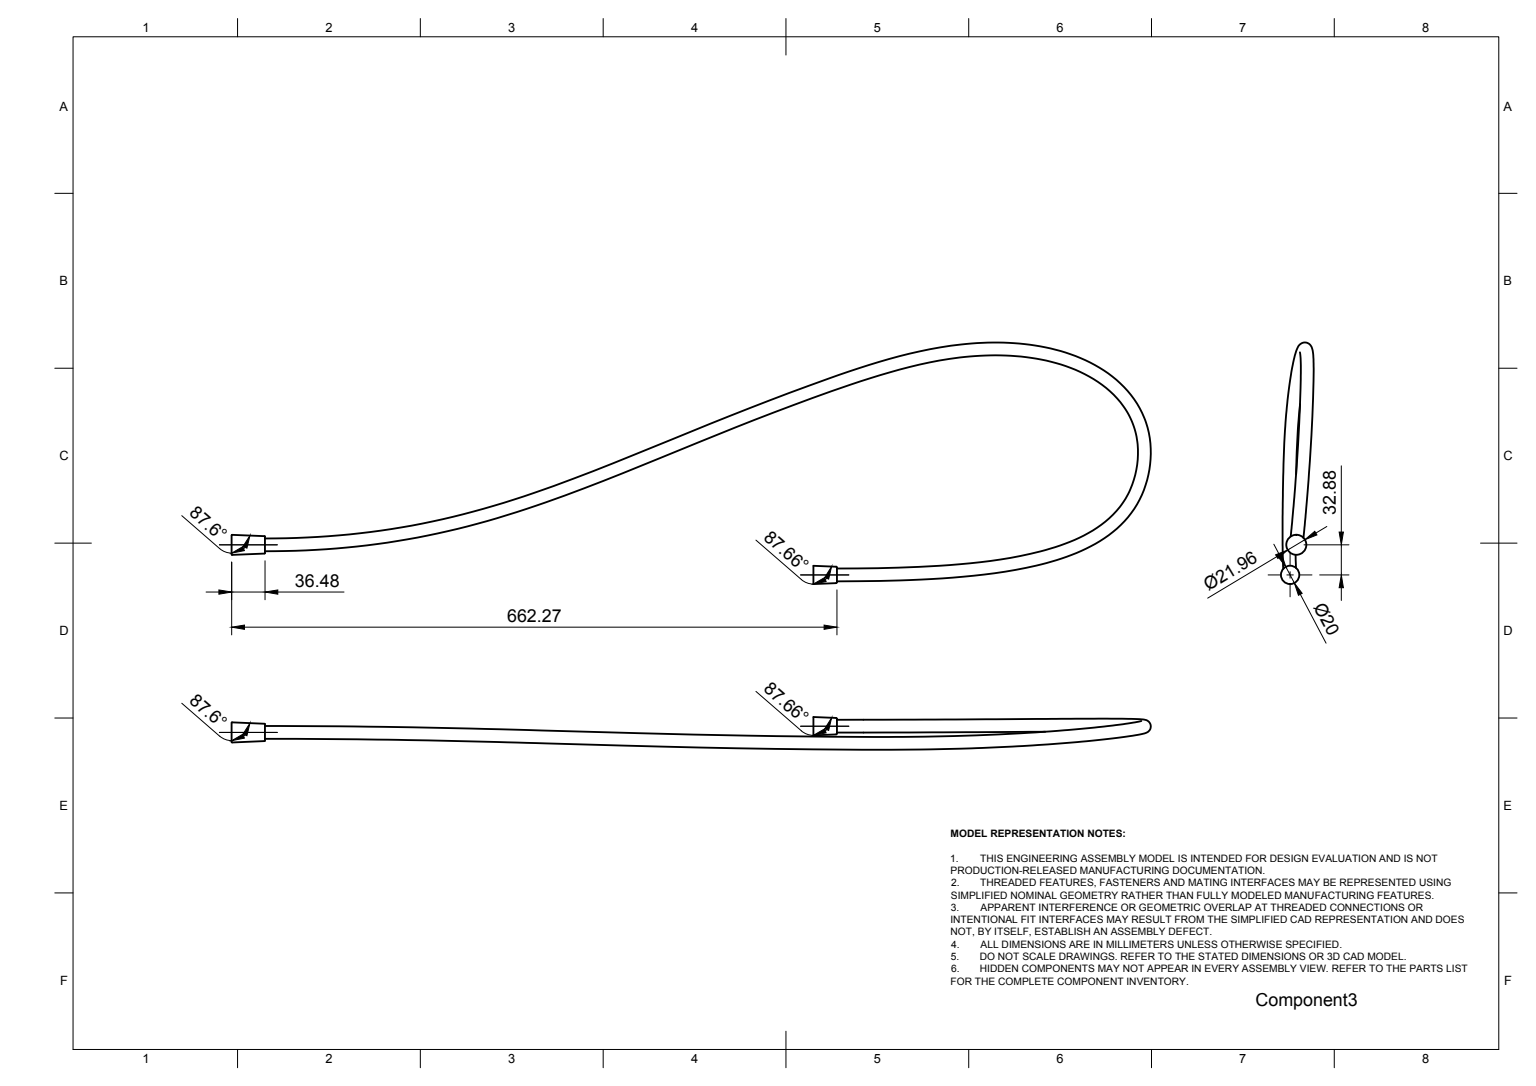
ISO-10303-21;
HEADER;
/* Generated by software containing ST-Developer
 * from STEP Tools, Inc. (www.steptools.com) 
 */

FILE_DESCRIPTION(
/* description */ ('STEP AP214'),
/* implementation_level */ '2;1');

FILE_NAME(
/* name */ 'Component3.step',
/* time_stamp */ '2026-10-06T11:02:40-07:00',
/* author */ (''),
/* organization */ (''),
/* preprocessor_version */ 'ST-DEVELOPER v20.2',
/* originating_system */ 'Autodesk Translation Framework v15.15.0.0',
/* authorisation */ '');

FILE_SCHEMA (('AUTOMOTIVE_DESIGN { 1 0 10303 214 3 1 1 }'));
ENDSEC;

DATA;
#10=MECHANICAL_DESIGN_GEOMETRIC_PRESENTATION_REPRESENTATION('',(#2938),#130910);
#76=CONICAL_SURFACE('',#48147,9.47320447306899,0.0418325464020223);
#77=CONICAL_SURFACE('',#48154,8.94802844775792,0.0407936828678657);
#715=FACE_BOUND('',#14926,.T.);
#716=FACE_BOUND('',#14930,.T.);
#1605=(
BOUNDED_SURFACE()
B_SPLINE_SURFACE(3,3,((#85020,#85021,#85022,#85023,#85024,#85025,#85026,
#85027,#85028,#85029,#85030,#85031,#85032,#85033,#85034,#85035,#85036,#85037,
#85038,#85039,#85040,#85041,#85042,#85043,#85044,#85045,#85046,#85047,#85048,
#85049,#85050,#85051,#85052,#85053,#85054,#85055,#85056,#85057,#85058,#85059,
#85060,#85061,#85062,#85063,#85064,#85065,#85066,#85067,#85068,#85069,#85070,
#85071,#85072,#85073),(#85074,#85075,#85076,#85077,#85078,#85079,#85080,
#85081,#85082,#85083,#85084,#85085,#85086,#85087,#85088,#85089,#85090,#85091,
#85092,#85093,#85094,#85095,#85096,#85097,#85098,#85099,#85100,#85101,#85102,
#85103,#85104,#85105,#85106,#85107,#85108,#85109,#85110,#85111,#85112,#85113,
#85114,#85115,#85116,#85117,#85118,#85119,#85120,#85121,#85122,#85123,#85124,
#85125,#85126,#85127),(#85128,#85129,#85130,#85131,#85132,#85133,#85134,
#85135,#85136,#85137,#85138,#85139,#85140,#85141,#85142,#85143,#85144,#85145,
#85146,#85147,#85148,#85149,#85150,#85151,#85152,#85153,#85154,#85155,#85156,
#85157,#85158,#85159,#85160,#85161,#85162,#85163,#85164,#85165,#85166,#85167,
#85168,#85169,#85170,#85171,#85172,#85173,#85174,#85175,#85176,#85177,#85178,
#85179,#85180,#85181),(#85182,#85183,#85184,#85185,#85186,#85187,#85188,
#85189,#85190,#85191,#85192,#85193,#85194,#85195,#85196,#85197,#85198,#85199,
#85200,#85201,#85202,#85203,#85204,#85205,#85206,#85207,#85208,#85209,#85210,
#85211,#85212,#85213,#85214,#85215,#85216,#85217,#85218,#85219,#85220,#85221,
#85222,#85223,#85224,#85225,#85226,#85227,#85228,#85229,#85230,#85231,#85232,
#85233,#85234,#85235),(#85236,#85237,#85238,#85239,#85240,#85241,#85242,
#85243,#85244,#85245,#85246,#85247,#85248,#85249,#85250,#85251,#85252,#85253,
#85254,#85255,#85256,#85257,#85258,#85259,#85260,#85261,#85262,#85263,#85264,
#85265,#85266,#85267,#85268,#85269,#85270,#85271,#85272,#85273,#85274,#85275,
#85276,#85277,#85278,#85279,#85280,#85281,#85282,#85283,#85284,#85285,#85286,
#85287,#85288,#85289),(#85290,#85291,#85292,#85293,#85294,#85295,#85296,
#85297,#85298,#85299,#85300,#85301,#85302,#85303,#85304,#85305,#85306,#85307,
#85308,#85309,#85310,#85311,#85312,#85313,#85314,#85315,#85316,#85317,#85318,
#85319,#85320,#85321,#85322,#85323,#85324,#85325,#85326,#85327,#85328,#85329,
#85330,#85331,#85332,#85333,#85334,#85335,#85336,#85337,#85338,#85339,#85340,
#85341,#85342,#85343),(#85344,#85345,#85346,#85347,#85348,#85349,#85350,
#85351,#85352,#85353,#85354,#85355,#85356,#85357,#85358,#85359,#85360,#85361,
#85362,#85363,#85364,#85365,#85366,#85367,#85368,#85369,#85370,#85371,#85372,
#85373,#85374,#85375,#85376,#85377,#85378,#85379,#85380,#85381,#85382,#85383,
#85384,#85385,#85386,#85387,#85388,#85389,#85390,#85391,#85392,#85393,#85394,
#85395,#85396,#85397)),.UNSPECIFIED.,.T.,.F.,.F.)
B_SPLINE_SURFACE_WITH_KNOTS((4,3,4),(4,2,2,2,2,2,2,2,2,2,2,2,2,2,2,2,2,
2,2,2,2,2,2,2,2,2,4),(0.,0.5,1.),(0.,0.00855967103632646,0.0171193420726529,
0.0342386841453058,0.0684773682906117,0.136954736581223,0.171193420726529,
0.205432104871835,0.239670789017141,0.273909473162447,0.302569805907928,
0.316899972280669,0.324065055467039,0.33123013865341,0.358116418237434,
0.385002697821458,0.438775256989507,0.492547816157555,0.546320375325604,
0.555016077087237,0.563711778848869,0.581103182372135,0.615885989418665,
0.711914492063999,0.807942994709333,0.903971497354666,1.),.UNSPECIFIED.)
GEOMETRIC_REPRESENTATION_ITEM()
RATIONAL_B_SPLINE_SURFACE(((1.,1.,1.,1.,1.,1.,1.,1.,1.,1.,1.,1.,1.,1.,1.,
1.,1.,1.,1.,1.,1.,1.,1.,1.,1.,1.,1.,1.,1.,1.,1.,1.,1.,1.,1.,1.,1.,1.,1.,
1.,1.,1.,1.,1.,1.,1.,1.,1.,1.,1.,1.,1.,1.,1.),(0.333333333333333,0.333333333333333,
0.333333333333333,0.333333333333333,0.333333333333333,0.333333333333333,
0.333333333333333,0.333333333333333,0.333333333333333,0.333333333333333,
0.333333333333333,0.333333333333333,0.333333333333333,0.333333333333333,
0.333333333333333,0.333333333333333,0.333333333333333,0.333333333333333,
0.333333333333333,0.333333333333333,0.333333333333333,0.333333333333333,
0.333333333333333,0.333333333333333,0.333333333333333,0.333333333333333,
0.333333333333333,0.333333333333333,0.333333333333333,0.333333333333333,
0.333333333333333,0.333333333333333,0.333333333333333,0.333333333333333,
0.333333333333333,0.333333333333333,0.333333333333333,0.333333333333333,
0.333333333333333,0.333333333333333,0.333333333333333,0.333333333333333,
0.333333333333333,0.333333333333333,0.333333333333333,0.333333333333333,
0.333333333333333,0.333333333333333,0.333333333333333,0.333333333333333,
0.333333333333333,0.333333333333333,0.333333333333333,0.333333333333333),
(0.333333333333333,0.333333333333333,0.333333333333333,0.333333333333333,
0.333333333333333,0.333333333333333,0.333333333333333,0.333333333333333,
0.333333333333333,0.333333333333333,0.333333333333333,0.333333333333333,
0.333333333333333,0.333333333333333,0.333333333333333,0.333333333333333,
0.333333333333333,0.333333333333333,0.333333333333333,0.333333333333333,
0.333333333333333,0.333333333333333,0.333333333333333,0.333333333333333,
0.333333333333333,0.333333333333333,0.333333333333333,0.333333333333333,
0.333333333333333,0.333333333333333,0.333333333333333,0.333333333333333,
0.333333333333333,0.333333333333333,0.333333333333333,0.333333333333333,
0.333333333333333,0.333333333333333,0.333333333333333,0.333333333333333,
0.333333333333333,0.333333333333333,0.333333333333333,0.333333333333333,
0.333333333333333,0.333333333333333,0.333333333333333,0.333333333333333,
0.333333333333333,0.333333333333333,0.333333333333333,0.333333333333333,
0.333333333333333,0.333333333333333),(1.,1.,1.,1.,1.,1.,1.,1.,1.,1.,1.,
1.,1.,1.,1.,1.,1.,1.,1.,1.,1.,1.,1.,1.,1.,1.,1.,1.,1.,1.,1.,1.,1.,1.,1.,
1.,1.,1.,1.,1.,1.,1.,1.,1.,1.,1.,1.,1.,1.,1.,1.,1.,1.,1.),(0.333333333333333,
0.333333333333333,0.333333333333333,0.333333333333333,0.333333333333333,
0.333333333333333,0.333333333333333,0.333333333333333,0.333333333333333,
0.333333333333333,0.333333333333333,0.333333333333333,0.333333333333333,
0.333333333333333,0.333333333333333,0.333333333333333,0.333333333333333,
0.333333333333333,0.333333333333333,0.333333333333333,0.333333333333333,
0.333333333333333,0.333333333333333,0.333333333333333,0.333333333333333,
0.333333333333333,0.333333333333333,0.333333333333333,0.333333333333333,
0.333333333333333,0.333333333333333,0.333333333333333,0.333333333333333,
0.333333333333333,0.333333333333333,0.333333333333333,0.333333333333333,
0.333333333333333,0.333333333333333,0.333333333333333,0.333333333333333,
0.333333333333333,0.333333333333333,0.333333333333333,0.333333333333333,
0.333333333333333,0.333333333333333,0.333333333333333,0.333333333333333,
0.333333333333333,0.333333333333333,0.333333333333333,0.333333333333333,
0.333333333333333),(0.333333333333333,0.333333333333333,0.333333333333333,
0.333333333333333,0.333333333333333,0.333333333333333,0.333333333333333,
0.333333333333333,0.333333333333333,0.333333333333333,0.333333333333333,
0.333333333333333,0.333333333333333,0.333333333333333,0.333333333333333,
0.333333333333333,0.333333333333333,0.333333333333333,0.333333333333333,
0.333333333333333,0.333333333333333,0.333333333333333,0.333333333333333,
0.333333333333333,0.333333333333333,0.333333333333333,0.333333333333333,
0.333333333333333,0.333333333333333,0.333333333333333,0.333333333333333,
0.333333333333333,0.333333333333333,0.333333333333333,0.333333333333333,
0.333333333333333,0.333333333333333,0.333333333333333,0.333333333333333,
0.333333333333333,0.333333333333333,0.333333333333333,0.333333333333333,
0.333333333333333,0.333333333333333,0.333333333333333,0.333333333333333,
0.333333333333333,0.333333333333333,0.333333333333333,0.333333333333333,
0.333333333333333,0.333333333333333,0.333333333333333),(1.,1.,1.,1.,1.,
1.,1.,1.,1.,1.,1.,1.,1.,1.,1.,1.,1.,1.,1.,1.,1.,1.,1.,1.,1.,1.,1.,1.,1.,
1.,1.,1.,1.,1.,1.,1.,1.,1.,1.,1.,1.,1.,1.,1.,1.,1.,1.,1.,1.,1.,1.,1.,1.,
1.)))
REPRESENTATION_ITEM('')
SURFACE()
);
#1606=(
BOUNDED_SURFACE()
B_SPLINE_SURFACE(3,3,((#85525,#85526,#85527,#85528,#85529,#85530,#85531,
#85532,#85533,#85534,#85535,#85536,#85537,#85538,#85539,#85540,#85541,#85542,
#85543,#85544,#85545,#85546,#85547,#85548,#85549,#85550,#85551,#85552,#85553,
#85554,#85555,#85556,#85557,#85558,#85559,#85560,#85561,#85562,#85563,#85564,
#85565,#85566,#85567,#85568,#85569,#85570,#85571,#85572,#85573,#85574,#85575,
#85576,#85577,#85578),(#85579,#85580,#85581,#85582,#85583,#85584,#85585,
#85586,#85587,#85588,#85589,#85590,#85591,#85592,#85593,#85594,#85595,#85596,
#85597,#85598,#85599,#85600,#85601,#85602,#85603,#85604,#85605,#85606,#85607,
#85608,#85609,#85610,#85611,#85612,#85613,#85614,#85615,#85616,#85617,#85618,
#85619,#85620,#85621,#85622,#85623,#85624,#85625,#85626,#85627,#85628,#85629,
#85630,#85631,#85632),(#85633,#85634,#85635,#85636,#85637,#85638,#85639,
#85640,#85641,#85642,#85643,#85644,#85645,#85646,#85647,#85648,#85649,#85650,
#85651,#85652,#85653,#85654,#85655,#85656,#85657,#85658,#85659,#85660,#85661,
#85662,#85663,#85664,#85665,#85666,#85667,#85668,#85669,#85670,#85671,#85672,
#85673,#85674,#85675,#85676,#85677,#85678,#85679,#85680,#85681,#85682,#85683,
#85684,#85685,#85686),(#85687,#85688,#85689,#85690,#85691,#85692,#85693,
#85694,#85695,#85696,#85697,#85698,#85699,#85700,#85701,#85702,#85703,#85704,
#85705,#85706,#85707,#85708,#85709,#85710,#85711,#85712,#85713,#85714,#85715,
#85716,#85717,#85718,#85719,#85720,#85721,#85722,#85723,#85724,#85725,#85726,
#85727,#85728,#85729,#85730,#85731,#85732,#85733,#85734,#85735,#85736,#85737,
#85738,#85739,#85740),(#85741,#85742,#85743,#85744,#85745,#85746,#85747,
#85748,#85749,#85750,#85751,#85752,#85753,#85754,#85755,#85756,#85757,#85758,
#85759,#85760,#85761,#85762,#85763,#85764,#85765,#85766,#85767,#85768,#85769,
#85770,#85771,#85772,#85773,#85774,#85775,#85776,#85777,#85778,#85779,#85780,
#85781,#85782,#85783,#85784,#85785,#85786,#85787,#85788,#85789,#85790,#85791,
#85792,#85793,#85794),(#85795,#85796,#85797,#85798,#85799,#85800,#85801,
#85802,#85803,#85804,#85805,#85806,#85807,#85808,#85809,#85810,#85811,#85812,
#85813,#85814,#85815,#85816,#85817,#85818,#85819,#85820,#85821,#85822,#85823,
#85824,#85825,#85826,#85827,#85828,#85829,#85830,#85831,#85832,#85833,#85834,
#85835,#85836,#85837,#85838,#85839,#85840,#85841,#85842,#85843,#85844,#85845,
#85846,#85847,#85848),(#85849,#85850,#85851,#85852,#85853,#85854,#85855,
#85856,#85857,#85858,#85859,#85860,#85861,#85862,#85863,#85864,#85865,#85866,
#85867,#85868,#85869,#85870,#85871,#85872,#85873,#85874,#85875,#85876,#85877,
#85878,#85879,#85880,#85881,#85882,#85883,#85884,#85885,#85886,#85887,#85888,
#85889,#85890,#85891,#85892,#85893,#85894,#85895,#85896,#85897,#85898,#85899,
#85900,#85901,#85902)),.UNSPECIFIED.,.T.,.F.,.F.)
B_SPLINE_SURFACE_WITH_KNOTS((4,3,4),(4,2,2,2,2,2,2,2,2,2,2,2,2,2,2,2,2,
2,2,2,2,2,2,2,2,2,4),(0.,0.5,1.),(0.,0.00855967103632646,0.0171193420726529,
0.0342386841453058,0.0684773682906117,0.136954736581223,0.171193420726529,
0.205432104871835,0.239670789017141,0.273909473162447,0.302569805907928,
0.316899972280669,0.324065055467039,0.33123013865341,0.358116418237434,
0.385002697821458,0.438775256989507,0.492547816157555,0.546320375325604,
0.555016077087237,0.563711778848869,0.581103182372135,0.615885989418665,
0.711914492063999,0.807942994709333,0.903971497354666,1.),.UNSPECIFIED.)
GEOMETRIC_REPRESENTATION_ITEM()
RATIONAL_B_SPLINE_SURFACE(((1.,1.,1.,1.,1.,1.,1.,1.,1.,1.,1.,1.,1.,1.,1.,
1.,1.,1.,1.,1.,1.,1.,1.,1.,1.,1.,1.,1.,1.,1.,1.,1.,1.,1.,1.,1.,1.,1.,1.,
1.,1.,1.,1.,1.,1.,1.,1.,1.,1.,1.,1.,1.,1.,1.),(0.333333333333333,0.333333333333333,
0.333333333333333,0.333333333333333,0.333333333333333,0.333333333333333,
0.333333333333333,0.333333333333333,0.333333333333333,0.333333333333333,
0.333333333333333,0.333333333333333,0.333333333333333,0.333333333333333,
0.333333333333333,0.333333333333333,0.333333333333333,0.333333333333333,
0.333333333333333,0.333333333333333,0.333333333333333,0.333333333333333,
0.333333333333333,0.333333333333333,0.333333333333333,0.333333333333333,
0.333333333333333,0.333333333333333,0.333333333333333,0.333333333333333,
0.333333333333333,0.333333333333333,0.333333333333333,0.333333333333333,
0.333333333333333,0.333333333333333,0.333333333333333,0.333333333333333,
0.333333333333333,0.333333333333333,0.333333333333333,0.333333333333333,
0.333333333333333,0.333333333333333,0.333333333333333,0.333333333333333,
0.333333333333333,0.333333333333333,0.333333333333333,0.333333333333333,
0.333333333333333,0.333333333333333,0.333333333333333,0.333333333333333),
(0.333333333333333,0.333333333333333,0.333333333333333,0.333333333333333,
0.333333333333333,0.333333333333333,0.333333333333333,0.333333333333333,
0.333333333333333,0.333333333333333,0.333333333333333,0.333333333333333,
0.333333333333333,0.333333333333333,0.333333333333333,0.333333333333333,
0.333333333333333,0.333333333333333,0.333333333333333,0.333333333333333,
0.333333333333333,0.333333333333333,0.333333333333333,0.333333333333333,
0.333333333333333,0.333333333333333,0.333333333333333,0.333333333333333,
0.333333333333333,0.333333333333333,0.333333333333333,0.333333333333333,
0.333333333333333,0.333333333333333,0.333333333333333,0.333333333333333,
0.333333333333333,0.333333333333333,0.333333333333333,0.333333333333333,
0.333333333333333,0.333333333333333,0.333333333333333,0.333333333333333,
0.333333333333333,0.333333333333333,0.333333333333333,0.333333333333333,
0.333333333333333,0.333333333333333,0.333333333333333,0.333333333333333,
0.333333333333333,0.333333333333333),(1.,1.,1.,1.,1.,1.,1.,1.,1.,1.,1.,
1.,1.,1.,1.,1.,1.,1.,1.,1.,1.,1.,1.,1.,1.,1.,1.,1.,1.,1.,1.,1.,1.,1.,1.,
1.,1.,1.,1.,1.,1.,1.,1.,1.,1.,1.,1.,1.,1.,1.,1.,1.,1.,1.),(0.333333333333333,
0.333333333333333,0.333333333333333,0.333333333333333,0.333333333333333,
0.333333333333333,0.333333333333333,0.333333333333333,0.333333333333333,
0.333333333333333,0.333333333333333,0.333333333333333,0.333333333333333,
0.333333333333333,0.333333333333333,0.333333333333333,0.333333333333333,
0.333333333333333,0.333333333333333,0.333333333333333,0.333333333333333,
0.333333333333333,0.333333333333333,0.333333333333333,0.333333333333333,
0.333333333333333,0.333333333333333,0.333333333333333,0.333333333333333,
0.333333333333333,0.333333333333333,0.333333333333333,0.333333333333333,
0.333333333333333,0.333333333333333,0.333333333333333,0.333333333333333,
0.333333333333333,0.333333333333333,0.333333333333333,0.333333333333333,
0.333333333333333,0.333333333333333,0.333333333333333,0.333333333333333,
0.333333333333333,0.333333333333333,0.333333333333333,0.333333333333333,
0.333333333333333,0.333333333333333,0.333333333333333,0.333333333333333,
0.333333333333333),(0.333333333333333,0.333333333333333,0.333333333333333,
0.333333333333333,0.333333333333333,0.333333333333333,0.333333333333333,
0.333333333333333,0.333333333333333,0.333333333333333,0.333333333333333,
0.333333333333333,0.333333333333333,0.333333333333333,0.333333333333333,
0.333333333333333,0.333333333333333,0.333333333333333,0.333333333333333,
0.333333333333333,0.333333333333333,0.333333333333333,0.333333333333333,
0.333333333333333,0.333333333333333,0.333333333333333,0.333333333333333,
0.333333333333333,0.333333333333333,0.333333333333333,0.333333333333333,
0.333333333333333,0.333333333333333,0.333333333333333,0.333333333333333,
0.333333333333333,0.333333333333333,0.333333333333333,0.333333333333333,
0.333333333333333,0.333333333333333,0.333333333333333,0.333333333333333,
0.333333333333333,0.333333333333333,0.333333333333333,0.333333333333333,
0.333333333333333,0.333333333333333,0.333333333333333,0.333333333333333,
0.333333333333333,0.333333333333333,0.333333333333333),(1.,1.,1.,1.,1.,
1.,1.,1.,1.,1.,1.,1.,1.,1.,1.,1.,1.,1.,1.,1.,1.,1.,1.,1.,1.,1.,1.,1.,1.,
1.,1.,1.,1.,1.,1.,1.,1.,1.,1.,1.,1.,1.,1.,1.,1.,1.,1.,1.,1.,1.,1.,1.,1.,
1.)))
REPRESENTATION_ITEM('')
SURFACE()
);
#2186=B_SPLINE_CURVE_WITH_KNOTS('',3,(#85402,#85403,#85404,#85405,#85406,
#85407,#85408,#85409,#85410,#85411,#85412,#85413,#85414,#85415,#85416,#85417,
#85418,#85419,#85420,#85421,#85422,#85423,#85424,#85425,#85426,#85427,#85428,
#85429,#85430,#85431,#85432,#85433,#85434,#85435,#85436,#85437,#85438,#85439,
#85440,#85441,#85442,#85443,#85444,#85445,#85446,#85447,#85448,#85449,#85450,
#85451,#85452,#85453,#85454,#85455),.UNSPECIFIED.,.F.,.F.,(4,2,2,2,2,2,
2,2,2,2,2,2,2,2,2,2,2,2,2,2,2,2,2,2,2,2,4),(0.,0.00855967103632646,0.0171193420726529,
0.0342386841453058,0.0684773682906117,0.136954736581223,0.171193420726529,
0.205432104871835,0.239670789017141,0.273909473162447,0.302569805907928,
0.316899972280669,0.324065055467039,0.33123013865341,0.358116418237434,
0.385002697821458,0.438775256989507,0.492547816157555,0.546320375325604,
0.555016077087237,0.563711778848869,0.581103182372135,0.615885989418665,
0.711914492063999,0.807942994709333,0.903971497354666,1.),.UNSPECIFIED.);
#2187=B_SPLINE_CURVE_WITH_KNOTS('',3,(#85458,#85459,#85460,#85461,#85462,
#85463,#85464,#85465,#85466,#85467,#85468,#85469,#85470,#85471,#85472,#85473,
#85474,#85475,#85476,#85477,#85478,#85479,#85480,#85481,#85482,#85483,#85484,
#85485,#85486,#85487,#85488,#85489,#85490,#85491,#85492,#85493,#85494,#85495,
#85496,#85497,#85498,#85499,#85500,#85501,#85502,#85503,#85504,#85505,#85506,
#85507,#85508,#85509,#85510,#85511),.UNSPECIFIED.,.F.,.F.,(4,2,2,2,2,2,
2,2,2,2,2,2,2,2,2,2,2,2,2,2,2,2,2,2,2,2,4),(0.,0.00855967103632646,0.0171193420726529,
0.0342386841453058,0.0684773682906117,0.136954736581223,0.171193420726529,
0.205432104871835,0.239670789017141,0.273909473162447,0.302569805907928,
0.316899972280669,0.324065055467039,0.33123013865341,0.358116418237434,
0.385002697821458,0.438775256989507,0.492547816157555,0.546320375325604,
0.555016077087237,0.563711778848869,0.581103182372135,0.615885989418665,
0.711914492063999,0.807942994709333,0.903971497354666,1.),.UNSPECIFIED.);
#2922=SHAPE_REPRESENTATION_RELATIONSHIP('SRR','None',#130944,#2930);
#2930=ADVANCED_BREP_SHAPE_REPRESENTATION('',(#2945),#130904);
#2938=STYLED_ITEM('',(#130991),#2945);
#2945=MANIFOLD_SOLID_BREP('Body1',#45452);
#3571=PLANE('',#48156);
#3572=PLANE('',#48157);
#3573=PLANE('',#48160);
#3574=PLANE('',#48161);
#5020=LINE('',#85019,#6794);
#5021=LINE('',#85521,#6795);
#6794=VECTOR('',#57507,9.47320447306899);
#6795=VECTOR('',#57524,8.94802844775792);
#10885=FACE_OUTER_BOUND('',#14918,.T.);
#10886=FACE_OUTER_BOUND('',#14919,.T.);
#10887=FACE_OUTER_BOUND('',#14920,.T.);
#10888=FACE_OUTER_BOUND('',#14921,.T.);
#10889=FACE_OUTER_BOUND('',#14922,.T.);
#10890=FACE_OUTER_BOUND('',#14923,.T.);
#10891=FACE_OUTER_BOUND('',#14924,.T.);
#10892=FACE_OUTER_BOUND('',#14925,.T.);
#10893=FACE_OUTER_BOUND('',#14927,.T.);
#10894=FACE_OUTER_BOUND('',#14928,.T.);
#10895=FACE_OUTER_BOUND('',#14929,.T.);
#14918=EDGE_LOOP('',(#35008,#35009,#35010,#35011,#35012));
#14919=EDGE_LOOP('',(#35013,#35014,#35015,#35016));
#14920=EDGE_LOOP('',(#35017,#35018,#35019,#35020,#35021));
#14921=EDGE_LOOP('',(#35022,#35023,#35024,#35025));
#14922=EDGE_LOOP('',(#35026,#35027,#35028,#35029));
#14923=EDGE_LOOP('',(#35030,#35031,#35032,#35033));
#14924=EDGE_LOOP('',(#35034));
#14925=EDGE_LOOP('',(#35035));
#14926=EDGE_LOOP('',(#35036,#35037));
#14927=EDGE_LOOP('',(#35038,#35039,#35040,#35041));
#14928=EDGE_LOOP('',(#35042));
#14929=EDGE_LOOP('',(#35043));
#14930=EDGE_LOOP('',(#35044,#35045));
#18957=CIRCLE('',#48139,10.9781962809611);
#18958=CIRCLE('',#48140,10.9781962809611);
#18959=CIRCLE('',#48141,0.5);
#18960=CIRCLE('',#48142,10.4786337076502);
#18961=CIRCLE('',#48144,9.49325771931311);
#18962=CIRCLE('',#48145,0.5);
#18963=CIRCLE('',#48146,8.99369514600215);
#18964=CIRCLE('',#48148,6.99999999999999);
#18965=CIRCLE('',#48149,6.99999999999999);
#18966=CIRCLE('',#48151,8.98718018777775);
#18967=CIRCLE('',#48152,1.);
#18968=CIRCLE('',#48153,7.98801213467717);
#18969=CIRCLE('',#48155,10.);
#18970=CIRCLE('',#48158,6.99999999999999);
#18971=CIRCLE('',#48159,6.99999999999999);
#22203=VERTEX_POINT('',#85005);
#22204=VERTEX_POINT('',#85006);
#22205=VERTEX_POINT('',#85009);
#22206=VERTEX_POINT('',#85013);
#22207=VERTEX_POINT('',#85015);
#22208=VERTEX_POINT('',#85398);
#22209=VERTEX_POINT('',#85399);
#22210=VERTEX_POINT('',#85401);
#22211=VERTEX_POINT('',#85456);
#22212=VERTEX_POINT('',#85513);
#22213=VERTEX_POINT('',#85515);
#22214=VERTEX_POINT('',#85519);
#26848=EDGE_CURVE('',#22203,#22204,#18957,.T.);
#26849=EDGE_CURVE('',#22204,#22203,#18958,.T.);
#26850=EDGE_CURVE('',#22204,#22205,#18959,.T.);
#26851=EDGE_CURVE('',#22205,#22205,#18960,.T.);
#26852=EDGE_CURVE('',#22206,#22206,#18961,.T.);
#26853=EDGE_CURVE('',#22206,#22207,#18962,.T.);
#26854=EDGE_CURVE('',#22207,#22207,#18963,.T.);
#26855=EDGE_CURVE('',#22203,#22206,#5020,.T.);
#26856=EDGE_CURVE('',#22208,#22209,#18964,.T.);
#26857=EDGE_CURVE('',#22209,#22210,#2186,.T.);
#26858=EDGE_CURVE('',#22211,#22210,#18965,.T.);
#26859=EDGE_CURVE('',#22208,#22211,#2187,.T.);
#26860=EDGE_CURVE('',#22212,#22212,#18966,.T.);
#26861=EDGE_CURVE('',#22212,#22213,#18967,.T.);
#26862=EDGE_CURVE('',#22213,#22213,#18968,.T.);
#26863=EDGE_CURVE('',#22214,#22214,#18969,.T.);
#26864=EDGE_CURVE('',#22214,#22212,#5021,.T.);
#26865=EDGE_CURVE('',#22209,#22208,#18970,.T.);
#26866=EDGE_CURVE('',#22210,#22211,#18971,.T.);
#35008=ORIENTED_EDGE('',*,*,#26848,.F.);
#35009=ORIENTED_EDGE('',*,*,#26849,.F.);
#35010=ORIENTED_EDGE('',*,*,#26850,.T.);
#35011=ORIENTED_EDGE('',*,*,#26851,.F.);
#35012=ORIENTED_EDGE('',*,*,#26850,.F.);
#35013=ORIENTED_EDGE('',*,*,#26852,.F.);
#35014=ORIENTED_EDGE('',*,*,#26853,.T.);
#35015=ORIENTED_EDGE('',*,*,#26854,.F.);
#35016=ORIENTED_EDGE('',*,*,#26853,.F.);
#35017=ORIENTED_EDGE('',*,*,#26848,.T.);
#35018=ORIENTED_EDGE('',*,*,#26849,.T.);
#35019=ORIENTED_EDGE('',*,*,#26855,.T.);
#35020=ORIENTED_EDGE('',*,*,#26852,.T.);
#35021=ORIENTED_EDGE('',*,*,#26855,.F.);
#35022=ORIENTED_EDGE('',*,*,#26856,.T.);
#35023=ORIENTED_EDGE('',*,*,#26857,.T.);
#35024=ORIENTED_EDGE('',*,*,#26858,.F.);
#35025=ORIENTED_EDGE('',*,*,#26859,.F.);
#35026=ORIENTED_EDGE('',*,*,#26860,.F.);
#35027=ORIENTED_EDGE('',*,*,#26861,.T.);
#35028=ORIENTED_EDGE('',*,*,#26862,.F.);
#35029=ORIENTED_EDGE('',*,*,#26861,.F.);
#35030=ORIENTED_EDGE('',*,*,#26863,.F.);
#35031=ORIENTED_EDGE('',*,*,#26864,.T.);
#35032=ORIENTED_EDGE('',*,*,#26860,.T.);
#35033=ORIENTED_EDGE('',*,*,#26864,.F.);
#35034=ORIENTED_EDGE('',*,*,#26863,.T.);
#35035=ORIENTED_EDGE('',*,*,#26862,.T.);
#35036=ORIENTED_EDGE('',*,*,#26856,.F.);
#35037=ORIENTED_EDGE('',*,*,#26865,.F.);
#35038=ORIENTED_EDGE('',*,*,#26857,.F.);
#35039=ORIENTED_EDGE('',*,*,#26865,.T.);
#35040=ORIENTED_EDGE('',*,*,#26859,.T.);
#35041=ORIENTED_EDGE('',*,*,#26866,.F.);
#35042=ORIENTED_EDGE('',*,*,#26851,.T.);
#35043=ORIENTED_EDGE('',*,*,#26854,.T.);
#35044=ORIENTED_EDGE('',*,*,#26858,.T.);
#35045=ORIENTED_EDGE('',*,*,#26866,.T.);
#41960=TOROIDAL_SURFACE('',#48138,10.4786337076502,0.5);
#41961=TOROIDAL_SURFACE('',#48143,8.99369514600215,0.5);
#41962=TOROIDAL_SURFACE('',#48150,7.98801213467717,1.);
#43465=ADVANCED_FACE('',(#10885),#41960,.T.);
#43466=ADVANCED_FACE('',(#10886),#41961,.T.);
#43467=ADVANCED_FACE('',(#10887),#76,.T.);
#43468=ADVANCED_FACE('',(#10888),#1605,.T.);
#43469=ADVANCED_FACE('',(#10889),#41962,.T.);
#43470=ADVANCED_FACE('',(#10890),#77,.T.);
#43471=ADVANCED_FACE('',(#10891),#3571,.F.);
#43472=ADVANCED_FACE('',(#10892,#715),#3572,.F.);
#43473=ADVANCED_FACE('',(#10893),#1606,.T.);
#43474=ADVANCED_FACE('',(#10894),#3573,.F.);
#43475=ADVANCED_FACE('',(#10895,#716),#3574,.F.);
#45452=CLOSED_SHELL('',(#43465,#43466,#43467,#43468,#43469,#43470,#43471,
#43472,#43473,#43474,#43475));
#48137=AXIS2_PLACEMENT_3D('',#85003,#57485,#57486);
#48138=AXIS2_PLACEMENT_3D('',#85004,#57487,#57488);
#48139=AXIS2_PLACEMENT_3D('',#85007,#57489,#57490);
#48140=AXIS2_PLACEMENT_3D('',#85008,#57491,#57492);
#48141=AXIS2_PLACEMENT_3D('',#85010,#57493,#57494);
#48142=AXIS2_PLACEMENT_3D('',#85011,#57495,#57496);
#48143=AXIS2_PLACEMENT_3D('',#85012,#57497,#57498);
#48144=AXIS2_PLACEMENT_3D('',#85014,#57499,#57500);
#48145=AXIS2_PLACEMENT_3D('',#85016,#57501,#57502);
#48146=AXIS2_PLACEMENT_3D('',#85017,#57503,#57504);
#48147=AXIS2_PLACEMENT_3D('',#85018,#57505,#57506);
#48148=AXIS2_PLACEMENT_3D('',#85400,#57508,#57509);
#48149=AXIS2_PLACEMENT_3D('',#85457,#57510,#57511);
#48150=AXIS2_PLACEMENT_3D('',#85512,#57512,#57513);
#48151=AXIS2_PLACEMENT_3D('',#85514,#57514,#57515);
#48152=AXIS2_PLACEMENT_3D('',#85516,#57516,#57517);
#48153=AXIS2_PLACEMENT_3D('',#85517,#57518,#57519);
#48154=AXIS2_PLACEMENT_3D('',#85518,#57520,#57521);
#48155=AXIS2_PLACEMENT_3D('',#85520,#57522,#57523);
#48156=AXIS2_PLACEMENT_3D('',#85522,#57525,#57526);
#48157=AXIS2_PLACEMENT_3D('',#85523,#57527,#57528);
#48158=AXIS2_PLACEMENT_3D('',#85524,#57529,#57530);
#48159=AXIS2_PLACEMENT_3D('',#85903,#57531,#57532);
#48160=AXIS2_PLACEMENT_3D('',#85904,#57533,#57534);
#48161=AXIS2_PLACEMENT_3D('',#85905,#57535,#57536);
#57485=DIRECTION('axis',(0.,0.,1.));
#57486=DIRECTION('refdir',(1.,0.,0.));
#57487=DIRECTION('center_axis',(0.,-1.,0.));
#57488=DIRECTION('ref_axis',(0.,0.,-1.));
#57489=DIRECTION('center_axis',(0.,-1.,0.));
#57490=DIRECTION('ref_axis',(0.,0.,-1.));
#57491=DIRECTION('center_axis',(0.,-1.,0.));
#57492=DIRECTION('ref_axis',(0.,0.,-1.));
#57493=DIRECTION('center_axis',(-1.,0.,0.));
#57494=DIRECTION('ref_axis',(0.,0.,1.));
#57495=DIRECTION('center_axis',(0.,1.,0.));
#57496=DIRECTION('ref_axis',(0.,0.,-1.));
#57497=DIRECTION('center_axis',(0.,1.,0.));
#57498=DIRECTION('ref_axis',(0.,0.,1.));
#57499=DIRECTION('center_axis',(0.,1.,0.));
#57500=DIRECTION('ref_axis',(0.,0.,-1.));
#57501=DIRECTION('center_axis',(-1.,0.,0.));
#57502=DIRECTION('ref_axis',(0.,0.,-1.));
#57503=DIRECTION('center_axis',(0.,-1.,0.));
#57504=DIRECTION('ref_axis',(0.,0.,1.));
#57505=DIRECTION('center_axis',(0.,1.,0.));
#57506=DIRECTION('ref_axis',(0.,0.,1.));
#57507=DIRECTION('',(5.12151535729607E-18,-0.999125146621934,0.041820346575534));
#57508=DIRECTION('center_axis',(0.,-1.,0.));
#57509=DIRECTION('ref_axis',(0.,0.,-1.));
#57510=DIRECTION('center_axis',(8.61122783338974E-15,1.,9.154793709916E-16));
#57511=DIRECTION('ref_axis',(0.161066048973386,-4.83449910768251E-16,-0.986943629529115));
#57512=DIRECTION('center_axis',(0.,1.,0.));
#57513=DIRECTION('ref_axis',(0.,0.,1.));
#57514=DIRECTION('center_axis',(0.,1.,0.));
#57515=DIRECTION('ref_axis',(0.,0.,-1.));
#57516=DIRECTION('center_axis',(-1.,0.,0.));
#57517=DIRECTION('ref_axis',(0.,0.,-1.));
#57518=DIRECTION('center_axis',(0.,-1.,0.));
#57519=DIRECTION('ref_axis',(0.,0.,1.));
#57520=DIRECTION('center_axis',(0.,1.,0.));
#57521=DIRECTION('ref_axis',(0.,0.,1.));
#57522=DIRECTION('center_axis',(0.,1.,0.));
#57523=DIRECTION('ref_axis',(0.,0.,1.));
#57524=DIRECTION('',(4.99439982873439E-18,-0.999168053100577,0.0407823695143096));
#57525=DIRECTION('center_axis',(0.,-1.,0.));
#57526=DIRECTION('ref_axis',(0.,0.,-1.));
#57527=DIRECTION('center_axis',(0.,1.,0.));
#57528=DIRECTION('ref_axis',(0.,0.,1.));
#57529=DIRECTION('center_axis',(0.,-1.,0.));
#57530=DIRECTION('ref_axis',(0.,0.,-1.));
#57531=DIRECTION('center_axis',(8.61122783338974E-15,1.,9.154793709916E-16));
#57532=DIRECTION('ref_axis',(0.161066048973386,-4.83449910768251E-16,-0.986943629529115));
#57533=DIRECTION('center_axis',(0.,-1.,0.));
#57534=DIRECTION('ref_axis',(0.,0.,-1.));
#57535=DIRECTION('center_axis',(0.,1.,0.));
#57536=DIRECTION('ref_axis',(0.,0.,1.));
#85003=CARTESIAN_POINT('',(0.,0.,0.));
#85004=CARTESIAN_POINT('Origin',(52.8776183915471,639.625373764374,90.6087118617898));
#85005=CARTESIAN_POINT('',(52.8776183915471,639.604463591086,79.6305155808287));
#85006=CARTESIAN_POINT('',(52.8776183915471,639.604463591086,101.586908142751));
#85007=CARTESIAN_POINT('Origin',(52.8776183915471,639.604463591086,90.6087118617898));
#85008=CARTESIAN_POINT('Origin',(52.8776183915471,639.604463591086,90.6087118617898));
#85009=CARTESIAN_POINT('',(52.8776183915471,640.125373764374,101.08734556944));
#85010=CARTESIAN_POINT('Origin',(52.8776183915471,639.625373764374,101.08734556944));
#85011=CARTESIAN_POINT('Origin',(52.8776183915471,640.125373764374,90.6087118617898));
#85012=CARTESIAN_POINT('Origin',(52.8776183915471,604.14887537019,90.6087118617898));
#85013=CARTESIAN_POINT('',(52.8776183915471,604.127965196902,81.1154541424767));
#85014=CARTESIAN_POINT('Origin',(52.8776183915471,604.127965196902,90.6087118617898));
#85015=CARTESIAN_POINT('',(52.8776183915471,603.64887537019,81.6150167157877));
#85016=CARTESIAN_POINT('Origin',(52.8776183915471,604.14887537019,81.6150167157877));
#85017=CARTESIAN_POINT('Origin',(52.8776183915471,603.64887537019,90.6087118617898));
#85018=CARTESIAN_POINT('Origin',(52.8776183915471,603.64887537019,90.6087118617898));
#85019=CARTESIAN_POINT('',(52.8776183915471,603.64887537019,81.1355073887209));
#85020=CARTESIAN_POINT('Ctrl Pts',(20.,-22.143643036685,76.7830741855192));
#85021=CARTESIAN_POINT('Ctrl Pts',(20.,-27.8457920778109,76.7830741857566));
#85022=CARTESIAN_POINT('Ctrl Pts',(20.0165214330532,-33.485592853313,76.7809705517141));
#85023=CARTESIAN_POINT('Ctrl Pts',(20.0854446608167,-44.638917128667,76.7729088380163));
#85024=CARTESIAN_POINT('Ctrl Pts',(20.1238292955523,-50.1526654673148,76.7668988331685));
#85025=CARTESIAN_POINT('Ctrl Pts',(20.4301340697073,-66.5001303791202,76.743985515181));
#85026=CARTESIAN_POINT('Ctrl Pts',(20.7188936123879,-77.141599114471,76.7227141396145));
#85027=CARTESIAN_POINT('Ctrl Pts',(21.8028495683285,-108.277666955853,76.643040982027));
#85028=CARTESIAN_POINT('Ctrl Pts',(22.8522177208893,-127.983498586547,76.568779347995));
#85029=CARTESIAN_POINT('Ctrl Pts',(27.2962882348799,-183.793342140183,76.3120470559144));
#85030=CARTESIAN_POINT('Ctrl Pts',(31.9889018993299,-216.590007789356,76.0958804243854));
#85031=CARTESIAN_POINT('Ctrl Pts',(42.752586146367,-258.54916325461,75.8385782220632));
#85032=CARTESIAN_POINT('Ctrl Pts',(46.9602598342624,-271.329384640549,75.7640306692479));
#85033=CARTESIAN_POINT('Ctrl Pts',(56.7935789905011,-294.374861216214,75.6600037328577));
#85034=CARTESIAN_POINT('Ctrl Pts',(62.4190261651095,-304.639843280753,75.6305279269569));
#85035=CARTESIAN_POINT('Ctrl Pts',(75.2624672361846,-322.558676299804,75.6391115492116));
#85036=CARTESIAN_POINT('Ctrl Pts',(82.4798249428642,-330.212646288195,75.6771562180411));
#85037=CARTESIAN_POINT('Ctrl Pts',(98.6902707967944,-342.825622479896,75.8431732977935));
#85038=CARTESIAN_POINT('Ctrl Pts',(107.683690787476,-347.785594002476,75.9711317990764));
#85039=CARTESIAN_POINT('Ctrl Pts',(126.023069913222,-354.340138637006,76.3098567703564));
#85040=CARTESIAN_POINT('Ctrl Pts',(135.083207114917,-356.371635015224,76.501925570174));
#85041=CARTESIAN_POINT('Ctrl Pts',(148.924338523526,-357.668316903019,76.9207856483578));
#85042=CARTESIAN_POINT('Ctrl Pts',(153.579247220674,-357.810711475144,77.0819658816335));
#85043=CARTESIAN_POINT('Ctrl Pts',(160.521670574454,-357.554693148273,77.3648314770126));
#85044=CARTESIAN_POINT('Ctrl Pts',(162.82915793653,-357.391086631896,77.4659695920693));
#85045=CARTESIAN_POINT('Ctrl Pts',(167.413894984383,-356.901529412086,77.6834093931112));
#85046=CARTESIAN_POINT('Ctrl Pts',(169.690165914981,-356.571218959933,77.800168876217));
#85047=CARTESIAN_POINT('Ctrl Pts',(180.410587995582,-354.672149675074,78.3871286663314));
#85048=CARTESIAN_POINT('Ctrl Pts',(188.539471171489,-351.990508745272,78.9676971116917));
#85049=CARTESIAN_POINT('Ctrl Pts',(203.935932366808,-344.394636660447,80.2994244971851));
#85050=CARTESIAN_POINT('Ctrl Pts',(211.203510672235,-339.480369996828,81.0505889748358));
#85051=CARTESIAN_POINT('Ctrl Pts',(231.426270328895,-321.586439483533,83.4642765655722));
#85052=CARTESIAN_POINT('Ctrl Pts',(242.801650331,-305.454778835795,85.2871564557421));
#85053=CARTESIAN_POINT('Ctrl Pts',(259.787422523192,-265.857198323714,88.846412059781));
#85054=CARTESIAN_POINT('Ctrl Pts',(265.396961479631,-242.39170484102,90.582652202398));
#85055=CARTESIAN_POINT('Ctrl Pts',(269.303802179431,-189.217670775394,93.4513081720829));
#85056=CARTESIAN_POINT('Ctrl Pts',(267.601212650846,-159.509605592023,94.5836348018781));
#85057=CARTESIAN_POINT('Ctrl Pts',(260.488092878426,-122.007461671797,95.2483440922483));
#85058=CARTESIAN_POINT('Ctrl Pts',(259.365919995518,-116.723004281873,95.3235942479774));
#85059=CARTESIAN_POINT('Ctrl Pts',(256.932101050909,-106.048555274698,95.4495336771278));
#85060=CARTESIAN_POINT('Ctrl Pts',(255.614336154295,-100.659660585315,95.4992578713651));
#85061=CARTESIAN_POINT('Ctrl Pts',(251.40188561101,-84.3843231292077,95.6128833960036));
#85062=CARTESIAN_POINT('Ctrl Pts',(248.248043744655,-73.3892261805465,95.6412376442078));
#85063=CARTESIAN_POINT('Ctrl Pts',(238.097187851482,-40.3402024940961,95.6176286794984));
#85064=CARTESIAN_POINT('Ctrl Pts',(230.410833839506,-18.2225145274556,95.4569933696899));
#85065=CARTESIAN_POINT('Ctrl Pts',(201.530604066263,61.5570672312919,94.6440942086903));
#85066=CARTESIAN_POINT('Ctrl Pts',(180.38355994371,113.231534550229,93.6242109681347));
#85067=CARTESIAN_POINT('Ctrl Pts',(140.797124795906,209.938840593949,91.236348118932));
#85068=CARTESIAN_POINT('Ctrl Pts',(122.357793139117,254.971482304575,89.8683893074086));
#85069=CARTESIAN_POINT('Ctrl Pts',(90.7794276043238,345.543709944167,87.281854516083));
#85070=CARTESIAN_POINT('Ctrl Pts',(77.6398467041473,391.083508984014,86.0632256586685));
#85071=CARTESIAN_POINT('Ctrl Pts',(59.2526292615706,489.828486097094,84.2723560895427));
#85072=CARTESIAN_POINT('Ctrl Pts',(54.0050807366749,543.034307838934,83.7001064546653));
#85073=CARTESIAN_POINT('Ctrl Pts',(54.0050807343608,603.648875370191,83.7001064550861));
#85074=CARTESIAN_POINT('Ctrl Pts',(34.,-22.143643036685,76.7830741855191));
#85075=CARTESIAN_POINT('Ctrl Pts',(33.9999999999839,-27.818749567832,76.7830741857369));
#85076=CARTESIAN_POINT('Ctrl Pts',(34.0164436970964,-33.4297565255892,76.7809804490342));
#85077=CARTESIAN_POINT('Ctrl Pts',(34.0849877845006,-44.5217274543659,76.7729629323669));
#85078=CARTESIAN_POINT('Ctrl Pts',(34.1231742300284,-50.0028679006344,76.7389494577223));
#85079=CARTESIAN_POINT('Ctrl Pts',(34.4276899601393,-66.246853907463,76.8982463815691));
#85080=CARTESIAN_POINT('Ctrl Pts',(34.7126441433325,-76.8114792097519,77.0127755335157));
#85081=CARTESIAN_POINT('Ctrl Pts',(35.7801701648313,-107.689013837462,77.2436000455983));
#85082=CARTESIAN_POINT('Ctrl Pts',(36.8122807199099,-127.185635036684,77.3200887338452));
#85083=CARTESIAN_POINT('Ctrl Pts',(41.1733655791691,-182.212078558018,77.4363129347258));
#85084=CARTESIAN_POINT('Ctrl Pts',(45.7887675371877,-214.28465811726,77.3652387134946));
#85085=CARTESIAN_POINT('Ctrl Pts',(56.1071091638816,-254.559565379267,77.2809282374505));
#85086=CARTESIAN_POINT('Ctrl Pts',(60.1071507567796,-266.675138787952,77.2549720220375));
#85087=CARTESIAN_POINT('Ctrl Pts',(69.2672710615284,-288.157823623031,77.2351548953765));
#85088=CARTESIAN_POINT('Ctrl Pts',(74.4235442697514,-297.51883236657,77.241288185783));
#85089=CARTESIAN_POINT('Ctrl Pts',(85.8799878791956,-313.508885526083,77.3068472367312));
#85090=CARTESIAN_POINT('Ctrl Pts',(92.1662088124034,-320.140602612327,77.3659108227464));
#85091=CARTESIAN_POINT('Ctrl Pts',(106.074791507621,-330.965616389605,77.5558022149426));
#85092=CARTESIAN_POINT('Ctrl Pts',(113.704741593858,-335.180562056838,77.6863058336575));
#85093=CARTESIAN_POINT('Ctrl Pts',(129.547452308994,-340.84513890228,78.019344686732));
#85094=CARTESIAN_POINT('Ctrl Pts',(137.504622410254,-342.63348319117,78.1724169021146));
#85095=CARTESIAN_POINT('Ctrl Pts',(149.585403594227,-343.765248871106,78.5379883229279));
#85096=CARTESIAN_POINT('Ctrl Pts',(153.635968157751,-343.887687412075,78.6783580728553));
#85097=CARTESIAN_POINT('Ctrl Pts',(159.628436780843,-343.666700644404,78.9225120249749));
#85098=CARTESIAN_POINT('Ctrl Pts',(161.61206380368,-343.525732039158,79.0094845712665));
#85099=CARTESIAN_POINT('Ctrl Pts',(165.532545967561,-343.107103515031,79.1954129140516));
#85100=CARTESIAN_POINT('Ctrl Pts',(167.468098111069,-342.826090867219,79.3037431318874));
#85101=CARTESIAN_POINT('Ctrl Pts',(176.532101218951,-341.217569579924,79.6978427041489));
#85102=CARTESIAN_POINT('Ctrl Pts',(183.383375567806,-338.959436198211,80.1037808086076));
#85103=CARTESIAN_POINT('Ctrl Pts',(196.476071197198,-332.501375371133,81.0647133327792));
#85104=CARTESIAN_POINT('Ctrl Pts',(202.718744012329,-328.297008645753,81.6202751258499));
#85105=CARTESIAN_POINT('Ctrl Pts',(220.341909241066,-312.716811913614,83.4515942144793));
#85106=CARTESIAN_POINT('Ctrl Pts',(230.624134911047,-298.333852015906,84.8966292281925));
#85107=CARTESIAN_POINT('Ctrl Pts',(246.265932818144,-261.956042751922,87.7965104150377));
#85108=CARTESIAN_POINT('Ctrl Pts',(251.601872159868,-239.986217448384,89.2479470149237));
#85109=CARTESIAN_POINT('Ctrl Pts',(255.356970654638,-189.502920762821,91.6411093546763));
#85110=CARTESIAN_POINT('Ctrl Pts',(253.780180374585,-160.998128460726,92.5820596772374));
#85111=CARTESIAN_POINT('Ctrl Pts',(246.932276322894,-124.751374927772,93.0704364824261));
#85112=CARTESIAN_POINT('Ctrl Pts',(245.842235402124,-119.627034808441,93.1558629346225));
#85113=CARTESIAN_POINT('Ctrl Pts',(243.475097814891,-109.245042637674,93.2783520239457));
#85114=CARTESIAN_POINT('Ctrl Pts',(242.190038398626,-103.98905174219,93.3268821124474));
#85115=CARTESIAN_POINT('Ctrl Pts',(238.072169272926,-88.0791416638133,93.4379565165972));
#85116=CARTESIAN_POINT('Ctrl Pts',(234.976567368465,-77.2836801120869,93.4659513934413));
#85117=CARTESIAN_POINT('Ctrl Pts',(224.980111926361,-44.7373516402995,93.4427019766555));
#85118=CARTESIAN_POINT('Ctrl Pts',(217.369979234584,-22.8302137815567,93.2841181941716));
#85119=CARTESIAN_POINT('Ctrl Pts',(188.65251219865,56.4997474834766,92.4758003573277));
#85120=CARTESIAN_POINT('Ctrl Pts',(167.598367439946,107.953240075026,91.4612213775221));
#85121=CARTESIAN_POINT('Ctrl Pts',(128.017986339935,204.645755313006,89.0737264657378));
#85122=CARTESIAN_POINT('Ctrl Pts',(109.483389981347,249.892586601305,87.6997062527036));
#85123=CARTESIAN_POINT('Ctrl Pts',(77.5768324188997,341.406124610584,85.0862925379845));
#85124=CARTESIAN_POINT('Ctrl Pts',(64.215495896169,387.677233373842,83.8475365004758));
#85125=CARTESIAN_POINT('Ctrl Pts',(45.5165434104212,488.096320975175,82.0263070967131));
#85126=CARTESIAN_POINT('Ctrl Pts',(40.1878699233725,542.222624701163,81.4451817692483));
#85127=CARTESIAN_POINT('Ctrl Pts',(40.1878699209532,603.648875370192,81.4451817694587));
#85128=CARTESIAN_POINT('Ctrl Pts',(34.,-22.143643036685,90.7830741855191));
#85129=CARTESIAN_POINT('Ctrl Pts',(33.9999999999666,-27.822192816507,90.7830741857369));
#85130=CARTESIAN_POINT('Ctrl Pts',(34.0164537550708,-33.4365739834866,90.7809791784461));
#85131=CARTESIAN_POINT('Ctrl Pts',(34.0850387982778,-44.5351482419418,90.7729568888413));
#85132=CARTESIAN_POINT('Ctrl Pts',(34.1512904613084,-50.0190681308895,90.7390437618613));
#85133=CARTESIAN_POINT('Ctrl Pts',(34.2738860204776,-66.275150464231,90.8979005786987));
#85134=CARTESIAN_POINT('Ctrl Pts',(34.4233619248085,-76.8497861166896,91.0101176438938));
#85135=CARTESIAN_POINT('Ctrl Pts',(35.1819506943524,-107.760797693274,91.2321643624032));
#85136=CARTESIAN_POINT('Ctrl Pts',(36.0651110374872,-127.285189611952,91.3003474514556));
#85137=CARTESIAN_POINT('Ctrl Pts',(40.0636907101652,-182.413148706558,91.3930827017859));
#85138=CARTESIAN_POINT('Ctrl Pts',(44.5459926487259,-214.577066409288,91.3077501454067));
#85139=CARTESIAN_POINT('Ctrl Pts',(54.7471862739539,-255.049764636043,91.2063086160594));
#85140=CARTESIAN_POINT('Ctrl Pts',(58.7239589095343,-267.241778858765,91.1752276768338));
#85141=CARTESIAN_POINT('Ctrl Pts',(67.8755199829761,-288.900859668629,91.1462563801209));
#85142=CARTESIAN_POINT('Ctrl Pts',(73.0468995042606,-298.36236982239,91.148353067284));
#85143=CARTESIAN_POINT('Ctrl Pts',(84.5856302727223,-314.566486013887,91.2071810262364));
#85144=CARTESIAN_POINT('Ctrl Pts',(90.9403044324173,-321.311526658035,91.2635796420002));
#85145=CARTESIAN_POINT('Ctrl Pts',(105.034746410925,-332.341129151079,91.4498791587053));
#85146=CARTESIAN_POINT('Ctrl Pts',(112.781438867057,-336.645409342233,91.5794836918854));
#85147=CARTESIAN_POINT('Ctrl Pts',(128.84379162978,-342.431310881406,91.9118603910799));
#85148=CARTESIAN_POINT('Ctrl Pts',(136.882331514546,-344.218066302979,92.06862737911));
#85149=CARTESIAN_POINT('Ctrl Pts',(149.042319260545,-345.35723535437,92.4365976867908));
#85150=CARTESIAN_POINT('Ctrl Pts',(153.113390074031,-345.479917353382,92.5777083987872));
#85151=CARTESIAN_POINT('Ctrl Pts',(159.128250624564,-345.258098659325,92.8227754054756));
#85152=CARTESIAN_POINT('Ctrl Pts',(161.117941330513,-345.116650646867,92.910018487043));
#85153=CARTESIAN_POINT('Ctrl Pts',(165.047777667848,-344.697015385526,93.0963913730309));
#85154=CARTESIAN_POINT('Ctrl Pts',(166.988577813154,-344.424194906112,93.2039800042653));
#85155=CARTESIAN_POINT('Ctrl Pts',(176.041505784734,-342.714803975454,93.6091367219815));
#85156=CARTESIAN_POINT('Ctrl Pts',(182.872054436279,-340.375843599256,94.0228196827679));
#85157=CARTESIAN_POINT('Ctrl Pts',(195.898526230413,-333.760723015434,94.9962526493361));
#85158=CARTESIAN_POINT('Ctrl Pts',(202.095700336024,-329.480194547591,95.5565589536698));
#85159=CARTESIAN_POINT('Ctrl Pts',(219.550609434862,-313.688603271014,97.3965554226442));
#85160=CARTESIAN_POINT('Ctrl Pts',(229.677969866178,-299.18923380383,98.8396419135539));
#85161=CARTESIAN_POINT('Ctrl Pts',(244.985390793916,-262.650450662216,101.721757946628));
#85162=CARTESIAN_POINT('Ctrl Pts',(250.143524864557,-240.635208284846,103.157649060994));
#85163=CARTESIAN_POINT('Ctrl Pts',(253.569471045668,-190.114279597768,105.514063707513));
#85164=CARTESIAN_POINT('Ctrl Pts',(251.841116264558,-161.616321569825,106.433990219553));
#85165=CARTESIAN_POINT('Ctrl Pts',(244.840413337758,-125.392448579826,106.898437331156));
#85166=CARTESIAN_POINT('Ctrl Pts',(243.762458422889,-120.265193874764,106.985804413879));
#85167=CARTESIAN_POINT('Ctrl Pts',(241.394977423079,-109.881694957916,107.108311299953));
#85168=CARTESIAN_POINT('Ctrl Pts',(240.109726258598,-104.624918046502,107.156848712739));
#85169=CARTESIAN_POINT('Ctrl Pts',(235.991218325549,-88.712539478757,107.267940365215));
#85170=CARTESIAN_POINT('Ctrl Pts',(232.89510653369,-77.9152866016949,107.295940488026));
#85171=CARTESIAN_POINT('Ctrl Pts',(222.896820184299,-45.3629955827255,107.272686881542));
#85172=CARTESIAN_POINT('Ctrl Pts',(215.28508460652,-23.4511547129986,107.114074507951));
#85173=CARTESIAN_POINT('Ctrl Pts',(186.559040616919,55.9024997794776,106.305515254125));
#85174=CARTESIAN_POINT('Ctrl Pts',(165.493582228552,107.38447679482,105.290480713943));
#85175=CARTESIAN_POINT('Ctrl Pts',(125.879107090836,204.160288949093,102.900929517052));
#85176=CARTESIAN_POINT('Ctrl Pts',(107.321611573323,249.462326772125,101.52526697662));
#85177=CARTESIAN_POINT('Ctrl Pts',(75.3707137533804,341.103048649986,98.9082216417973));
#85178=CARTESIAN_POINT('Ctrl Pts',(61.9890301742715,387.445708532525,97.6675820645533));
#85179=CARTESIAN_POINT('Ctrl Pts',(43.265762695917,487.995387928407,95.8439845955144));
#85180=CARTESIAN_POINT('Ctrl Pts',(37.9329452373243,542.179444956935,95.2623925830766));
#85181=CARTESIAN_POINT('Ctrl Pts',(37.9329452353258,603.648875370192,95.2623925828662));
#85182=CARTESIAN_POINT('Ctrl Pts',(20.,-22.143643036685,90.7830741855191));
#85183=CARTESIAN_POINT('Ctrl Pts',(20.0000000000198,-27.8492353264858,90.7830741857566));
#85184=CARTESIAN_POINT('Ctrl Pts',(20.016531491053,-33.4924103112104,90.7809692811259));
#85185=CARTESIAN_POINT('Ctrl Pts',(20.0854956745684,-44.652337916243,90.7729027944908));
#85186=CARTESIAN_POINT('Ctrl Pts',(20.1519455268513,-50.1688656975699,90.7669931373075));
#85187=CARTESIAN_POINT('Ctrl Pts',(20.2763301300078,-66.5284269358881,90.7436397123106));
#85188=CARTESIAN_POINT('Ctrl Pts',(20.4296113938976,-77.1799060213726,90.7200562499926));
#85189=CARTESIAN_POINT('Ctrl Pts',(21.204630097782,-108.349450811737,90.6316052988318));
#85190=CARTESIAN_POINT('Ctrl Pts',(22.10504803841,-128.083053161685,90.5490380656054));
#85191=CARTESIAN_POINT('Ctrl Pts',(26.1866133659894,-183.994412288981,90.2688168229746));
#85192=CARTESIAN_POINT('Ctrl Pts',(30.746127010843,-216.882416081384,90.0383918562974));
#85193=CARTESIAN_POINT('Ctrl Pts',(41.3926632564519,-259.039362511386,89.7639586006721));
#85194=CARTESIAN_POINT('Ctrl Pts',(45.5770679869517,-271.896024711361,89.6842863240442));
#85195=CARTESIAN_POINT('Ctrl Pts',(55.4018279120142,-295.117897261812,89.5711052176021));
#85196=CARTESIAN_POINT('Ctrl Pts',(61.0423813996187,-305.483380736572,89.537592808458));
#85197=CARTESIAN_POINT('Ctrl Pts',(73.9681096297112,-323.616276787607,89.5394453387168));
#85198=CARTESIAN_POINT('Ctrl Pts',(81.2539205629141,-331.38357033419,89.574825037295));
#85199=CARTESIAN_POINT('Ctrl Pts',(97.6502257000617,-344.201135241083,89.7372502415561));
#85200=CARTESIAN_POINT('Ctrl Pts',(106.760388060712,-349.250441287872,89.8643096573043));
#85201=CARTESIAN_POINT('Ctrl Pts',(125.319409233977,-355.926310616132,90.2023724747043));
#85202=CARTESIAN_POINT('Ctrl Pts',(134.460916219209,-357.956218127161,90.3981360471693));
#85203=CARTESIAN_POINT('Ctrl Pts',(148.381254189844,-359.260303386218,90.8193950122208));
#85204=CARTESIAN_POINT('Ctrl Pts',(153.056669136986,-359.402941416322,90.9813162075653));
#85205=CARTESIAN_POINT('Ctrl Pts',(160.021484418159,-359.146091163259,91.2650948575132));
#85206=CARTESIAN_POINT('Ctrl Pts',(162.335035463347,-358.982005239573,91.3665035078458));
#85207=CARTESIAN_POINT('Ctrl Pts',(166.929126684686,-358.491441282613,91.5843878520904));
#85208=CARTESIAN_POINT('Ctrl Pts',(169.210645617082,-358.169322998826,91.7004057485949));
#85209=CARTESIAN_POINT('Ctrl Pts',(179.919992561305,-356.169384070604,92.298422684164));
#85210=CARTESIAN_POINT('Ctrl Pts',(188.028150039962,-353.406916146197,92.886735985852));
#85211=CARTESIAN_POINT('Ctrl Pts',(203.358387400023,-345.653984304867,94.2309638137419));
#85212=CARTESIAN_POINT('Ctrl Pts',(210.580466995992,-340.663555898792,94.9868728026557));
#85213=CARTESIAN_POINT('Ctrl Pts',(230.634970522565,-322.558230840682,97.4092377737371));
#85214=CARTESIAN_POINT('Ctrl Pts',(241.855485286281,-306.310160623718,99.2301691411035));
#85215=CARTESIAN_POINT('Ctrl Pts',(258.506880498815,-266.551606234007,102.771659591371));
#85216=CARTESIAN_POINT('Ctrl Pts',(263.93861418432,-243.040695677481,104.492354248469));
#85217=CARTESIAN_POINT('Ctrl Pts',(267.516302570461,-189.829029610341,107.32426252492));
#85218=CARTESIAN_POINT('Ctrl Pts',(265.662148540819,-160.127798701236,108.435565344194));
#85219=CARTESIAN_POINT('Ctrl Pts',(258.396229893289,-122.648535323832,109.076344940978));
#85220=CARTESIAN_POINT('Ctrl Pts',(257.286143016284,-117.361163348158,109.153535727234));
#85221=CARTESIAN_POINT('Ctrl Pts',(254.851980659096,-106.685207594979,109.279492953135));
#85222=CARTESIAN_POINT('Ctrl Pts',(253.534024014268,-101.295526889627,109.329224471656));
#85223=CARTESIAN_POINT('Ctrl Pts',(249.320934663633,-85.0177209441514,109.442867244621));
#85224=CARTESIAN_POINT('Ctrl Pts',(246.16658290972,-74.0208326701545,109.471226738793));
#85225=CARTESIAN_POINT('Ctrl Pts',(236.013896109739,-40.9658464365221,109.447613584385));
#85226=CARTESIAN_POINT('Ctrl Pts',(228.325939211598,-18.8434554588877,109.28694968347));
#85227=CARTESIAN_POINT('Ctrl Pts',(199.4371324841,60.9598195272659,108.473809105488));
#85228=CARTESIAN_POINT('Ctrl Pts',(178.278774731953,112.662771270022,107.453470304555));
#85229=CARTESIAN_POINT('Ctrl Pts',(138.658245547169,209.453374230036,105.063551170246));
#85230=CARTESIAN_POINT('Ctrl Pts',(120.196014730927,254.541222475395,103.693950031325));
#85231=CARTESIAN_POINT('Ctrl Pts',(88.5733089389711,345.240633983569,101.103783619896));
#85232=CARTESIAN_POINT('Ctrl Pts',(75.4133809825114,390.851984142697,99.8832712227459));
#85233=CARTESIAN_POINT('Ctrl Pts',(57.0018485468049,489.727553050326,98.090033588344));
#85234=CARTESIAN_POINT('Ctrl Pts',(51.7501560506267,542.991128087974,97.5173172684936));
#85235=CARTESIAN_POINT('Ctrl Pts',(51.7501560487334,603.648875370191,97.5173172684936));
#85236=CARTESIAN_POINT('Ctrl Pts',(6.,-22.143643036685,90.7830741855191));
#85237=CARTESIAN_POINT('Ctrl Pts',(6.00000000007298,-27.8762778364647,90.7830741857764));
#85238=CARTESIAN_POINT('Ctrl Pts',(6.01660922703522,-33.5482466389342,90.7809593838058));
#85239=CARTESIAN_POINT('Ctrl Pts',(6.08595255085911,-44.7695275905442,90.7728487001403));
#85240=CARTESIAN_POINT('Ctrl Pts',(6.15260059239406,-50.3186632642503,90.7949425127537));
#85241=CARTESIAN_POINT('Ctrl Pts',(6.27877423953789,-66.7817034075453,90.5893788459225));
#85242=CARTESIAN_POINT('Ctrl Pts',(6.43586086298679,-77.5100259260557,90.4299948560914));
#85243=CARTESIAN_POINT('Ctrl Pts',(7.22730950121153,-108.9381039302,90.0310462352604));
#85244=CARTESIAN_POINT('Ctrl Pts',(8.14498503933279,-128.880916711419,89.7977286797552));
#85245=CARTESIAN_POINT('Ctrl Pts',(12.3095360218137,-185.575675871405,89.1445509441633));
#85246=CARTESIAN_POINT('Ctrl Pts',(16.9462613729601,-219.18776575348,88.7690335671882));
#85247=CARTESIAN_POINT('Ctrl Pts',(28.0381402389499,-263.028960386728,88.3216085852849));
#85248=CARTESIAN_POINT('Ctrl Pts',(32.4301770643691,-276.550270563958,88.1933449712546));
#85249=CARTESIAN_POINT('Ctrl Pts',(42.9281358410523,-301.334934854994,87.9959540550834));
#85250=CARTESIAN_POINT('Ctrl Pts',(49.0378632949769,-312.604391650755,87.9268325496319));
#85251=CARTESIAN_POINT('Ctrl Pts',(63.3505889867002,-332.666067561327,87.8717096511972));
#85252=CARTESIAN_POINT('Ctrl Pts',(71.5675366934108,-341.455614010345,87.8860704325898));
#85253=CARTESIAN_POINT('Ctrl Pts',(90.2657049891989,-356.061141331087,88.024621324407));
#85254=CARTESIAN_POINT('Ctrl Pts',(100.739337254366,-361.85547323351,88.1491356227232));
#85255=CARTESIAN_POINT('Ctrl Pts',(121.795026838174,-369.421310350857,88.4928845583287));
#85256=CARTESIAN_POINT('Ctrl Pts',(132.039500923872,-371.694369951344,88.7276447152287));
#85257=CARTESIAN_POINT('Ctrl Pts',(147.720189119143,-373.163371418067,89.2021923376507));
#85258=CARTESIAN_POINT('Ctrl Pts',(152.999948199941,-373.325965479262,89.3849240163435));
#85259=CARTESIAN_POINT('Ctrl Pts',(160.914718211754,-373.034083667193,89.7074143095509));
#85260=CARTESIAN_POINT('Ctrl Pts',(163.552129596181,-372.84735983228,89.8229885286486));
#85261=CARTESIAN_POINT('Ctrl Pts',(168.810475701525,-372.285867179701,90.07238433115));
#85262=CARTESIAN_POINT('Ctrl Pts',(171.43271342101,-371.91445109154,90.1968314929245));
#85263=CARTESIAN_POINT('Ctrl Pts',(183.798479337875,-369.623964165754,90.9877086463466));
#85264=CARTESIAN_POINT('Ctrl Pts',(193.184245643645,-366.437988693138,91.7506522889361));
#85265=CARTESIAN_POINT('Ctrl Pts',(210.818248569633,-357.5472455943,93.4656749781478));
#85266=CARTESIAN_POINT('Ctrl Pts',(219.06523365596,-351.846917249993,94.4171866516416));
#85267=CARTESIAN_POINT('Ctrl Pts',(241.719331610269,-331.42785841035,97.42192012483));
#85268=CARTESIAN_POINT('Ctrl Pts',(254.033000706385,-313.431087443606,99.6206963686531));
#85269=CARTESIAN_POINT('Ctrl Pts',(272.028370203714,-270.452761805799,103.821561236115));
#85270=CARTESIAN_POINT('Ctrl Pts',(277.733703504083,-245.446183070117,105.827059435943));
#85271=CARTESIAN_POINT('Ctrl Pts',(281.463134095255,-189.543779622914,109.134461342326));
#85272=CARTESIAN_POINT('Ctrl Pts',(279.48318081708,-158.639275832648,110.437140468834));
#85273=CARTESIAN_POINT('Ctrl Pts',(271.952046448821,-119.904622067839,111.2542525508));
#85274=CARTESIAN_POINT('Ctrl Pts',(270.809827609678,-114.457132821552,111.321267040589));
#85275=CARTESIAN_POINT('Ctrl Pts',(268.308983895114,-103.488720232041,111.450674606317));
#85276=CARTESIAN_POINT('Ctrl Pts',(266.958321769937,-97.9661357327517,111.501600230574));
#85277=CARTESIAN_POINT('Ctrl Pts',(262.650651001717,-81.3229024095457,111.617794124028));
#85278=CARTESIAN_POINT('Ctrl Pts',(259.438059285751,-70.1263787386142,111.646512989559));
#85279=CARTESIAN_POINT('Ctrl Pts',(249.130972035179,-36.5686972903188,111.622540287227));
#85280=CARTESIAN_POINT('Ctrl Pts',(241.366793816677,-14.2357562047768,111.459824858988));
#85281=CARTESIAN_POINT('Ctrl Pts',(212.315224351282,66.0171392750542,110.64210295685));
#85282=CARTESIAN_POINT('Ctrl Pts',(191.063967235354,117.941065745225,109.616459895168));
#85283=CARTESIAN_POINT('Ctrl Pts',(151.437384003502,214.746459510979,107.22617282344));
#85284=CARTESIAN_POINT('Ctrl Pts',(133.070417888531,259.620118178664,105.86263308603));
#85285=CARTESIAN_POINT('Ctrl Pts',(101.775904124562,349.378219317153,103.299345597994));
#85286=CARTESIAN_POINT('Ctrl Pts',(88.8377317907513,394.25825975287,102.098960380939));
#85287=CARTESIAN_POINT('Ctrl Pts',(70.7379343976928,491.459718172245,100.336082581174));
#85288=CARTESIAN_POINT('Ctrl Pts',(65.5673668639291,543.802811219013,99.7722419539107));
#85289=CARTESIAN_POINT('Ctrl Pts',(65.567366862141,603.648875370191,99.772241954121));
#85290=CARTESIAN_POINT('Ctrl Pts',(6.,-22.143643036685,76.7830741855191));
#85291=CARTESIAN_POINT('Ctrl Pts',(6.00000000001608,-27.8728345877897,76.7830741857764));
#85292=CARTESIAN_POINT('Ctrl Pts',(6.01659916901003,-33.5414291810368,76.7809606543939));
#85293=CARTESIAN_POINT('Ctrl Pts',(6.08590153713278,-44.7561068029682,76.7728547436659));
#85294=CARTESIAN_POINT('Ctrl Pts',(6.12448436107623,-50.3024630339952,76.7948482086147));
#85295=CARTESIAN_POINT('Ctrl Pts',(6.43257817927521,-66.7534068507774,76.5897246487929));
#85296=CARTESIAN_POINT('Ctrl Pts',(6.72514308144325,-77.47171901919,76.4326527457133));
#85297=CARTESIAN_POINT('Ctrl Pts',(7.82552897182559,-108.866320074244,76.0424819184556));
#85298=CARTESIAN_POINT('Ctrl Pts',(8.89215472186884,-128.78136213641,75.8174699621448));
#85299=CARTESIAN_POINT('Ctrl Pts',(13.4192108905908,-185.374605722347,75.1877811771031));
#85300=CARTESIAN_POINT('Ctrl Pts',(18.189036261472,-218.895357461452,74.8265221352761));
#85301=CARTESIAN_POINT('Ctrl Pts',(29.3980631288525,-262.538761129952,74.3962282066761));
#85302=CARTESIAN_POINT('Ctrl Pts',(33.8133689117452,-275.983630493145,74.2730893164583));
#85303=CARTESIAN_POINT('Ctrl Pts',(44.3198869194738,-300.591898809396,74.0848525703389));
#85304=CARTESIAN_POINT('Ctrl Pts',(50.4145080604677,-311.760854194936,74.0197676681309));
#85305=CARTESIAN_POINT('Ctrl Pts',(64.6449465931735,-331.608467073524,73.9713758616919));
#85306=CARTESIAN_POINT('Ctrl Pts',(72.793441073325,-340.284689964064,73.9884016133359));
#85307=CARTESIAN_POINT('Ctrl Pts',(91.3057500859674,-354.685628570187,74.1305443806443));
#85308=CARTESIAN_POINT('Ctrl Pts',(101.662639981094,-360.390625948114,74.2559577644952));
#85309=CARTESIAN_POINT('Ctrl Pts',(122.498687517451,-367.835138371731,74.6003688539808));
#85310=CARTESIAN_POINT('Ctrl Pts',(132.66179181958,-370.109786839278,74.8314342382333));
#85311=CARTESIAN_POINT('Ctrl Pts',(148.263273452825,-371.571384934932,75.3035829737878));
#85312=CARTESIAN_POINT('Ctrl Pts',(153.522526283597,-371.733735538213,75.4855736904116));
#85313=CARTESIAN_POINT('Ctrl Pts',(161.414904368065,-371.442685652143,75.8071509290502));
#85314=CARTESIAN_POINT('Ctrl Pts',(164.04625206938,-371.256441224634,75.922454612872));
#85315=CARTESIAN_POINT('Ctrl Pts',(169.295244001206,-370.695955309142,76.1714058721708));
#85316=CARTESIAN_POINT('Ctrl Pts',(171.912233718893,-370.316347052647,76.2965946205466));
#85317=CARTESIAN_POINT('Ctrl Pts',(184.289074772213,-368.126729770224,77.0764146285139));
#85318=CARTESIAN_POINT('Ctrl Pts',(193.695566775172,-365.021581292332,77.8316134147758));
#85319=CARTESIAN_POINT('Ctrl Pts',(211.395793536418,-356.28789794976,79.5341356615909));
#85320=CARTESIAN_POINT('Ctrl Pts',(219.68827733214,-350.663731347904,80.4809028238217));
#85321=CARTESIAN_POINT('Ctrl Pts',(242.510631416724,-330.456067053452,83.4769589166651));
#85322=CARTESIAN_POINT('Ctrl Pts',(254.979165750953,-312.575705655683,85.6776836832917));
#85323=CARTESIAN_POINT('Ctrl Pts',(273.308912228241,-269.758353895505,89.8963137045242));
#85324=CARTESIAN_POINT('Ctrl Pts',(279.192050799395,-244.797192233655,91.9173573898723));
#85325=CARTESIAN_POINT('Ctrl Pts',(283.250633704224,-188.932420787966,95.2615069894894));
#85326=CARTESIAN_POINT('Ctrl Pts',(281.422244927106,-158.021082723321,96.5852099265189));
#85327=CARTESIAN_POINT('Ctrl Pts',(274.043909433957,-119.263548415822,97.4262517020704));
#85328=CARTESIAN_POINT('Ctrl Pts',(272.889604588913,-113.818973755306,97.4913255613324));
#85329=CARTESIAN_POINT('Ctrl Pts',(270.389104286926,-102.852067911723,97.6207153303099));
#85330=CARTESIAN_POINT('Ctrl Pts',(269.038633909964,-97.3302694284403,97.6716336302827));
#85331=CARTESIAN_POINT('Ctrl Pts',(264.731601949094,-80.689504594602,97.78781027541));
#85332=CARTESIAN_POINT('Ctrl Pts',(261.519520120845,-69.4947722490061,97.8165238949743));
#85333=CARTESIAN_POINT('Ctrl Pts',(251.214263776602,-35.9430533478927,97.7925553823412));
#85334=CARTESIAN_POINT('Ctrl Pts',(243.451688444427,-13.6148152733545,97.6298685452083));
#85335=CARTESIAN_POINT('Ctrl Pts',(214.408695933877,66.6143869791072,96.812388060053));
#85336=CARTESIAN_POINT('Ctrl Pts',(193.168752447473,118.509829025431,95.7872005587473));
#85337=CARTESIAN_POINT('Ctrl Pts',(153.576263251876,215.231925874893,93.3989697721262));
#85338=CARTESIAN_POINT('Ctrl Pts',(135.232196296888,260.050378007844,92.0370723621136));
#85339=CARTESIAN_POINT('Ctrl Pts',(103.982022789748,349.68129527775,89.4774164941815));
#85340=CARTESIAN_POINT('Ctrl Pts',(91.0641975121257,394.489784594186,88.2789148168611));
#85341=CARTESIAN_POINT('Ctrl Pts',(72.9887151127201,491.560651219013,86.5184050823723));
#85342=CARTESIAN_POINT('Ctrl Pts',(67.8222915499773,543.845990976705,85.9550311400823));
#85343=CARTESIAN_POINT('Ctrl Pts',(67.8222915477683,603.648875370191,85.9550311407135));
#85344=CARTESIAN_POINT('Ctrl Pts',(20.,-22.143643036685,76.7830741855192));
#85345=CARTESIAN_POINT('Ctrl Pts',(20.,-27.8457920778109,76.7830741857566));
#85346=CARTESIAN_POINT('Ctrl Pts',(20.0165214330532,-33.485592853313,76.7809705517141));
#85347=CARTESIAN_POINT('Ctrl Pts',(20.0854446608167,-44.638917128667,76.7729088380163));
#85348=CARTESIAN_POINT('Ctrl Pts',(20.1238292955523,-50.1526654673148,76.7668988331685));
#85349=CARTESIAN_POINT('Ctrl Pts',(20.4301340697073,-66.5001303791202,76.743985515181));
#85350=CARTESIAN_POINT('Ctrl Pts',(20.7188936123879,-77.141599114471,76.7227141396145));
#85351=CARTESIAN_POINT('Ctrl Pts',(21.8028495683285,-108.277666955853,76.643040982027));
#85352=CARTESIAN_POINT('Ctrl Pts',(22.8522177208893,-127.983498586547,76.568779347995));
#85353=CARTESIAN_POINT('Ctrl Pts',(27.2962882348799,-183.793342140183,76.3120470559144));
#85354=CARTESIAN_POINT('Ctrl Pts',(31.9889018993299,-216.590007789356,76.0958804243854));
#85355=CARTESIAN_POINT('Ctrl Pts',(42.752586146367,-258.54916325461,75.8385782220632));
#85356=CARTESIAN_POINT('Ctrl Pts',(46.9602598342624,-271.329384640549,75.7640306692479));
#85357=CARTESIAN_POINT('Ctrl Pts',(56.7935789905011,-294.374861216214,75.6600037328577));
#85358=CARTESIAN_POINT('Ctrl Pts',(62.4190261651095,-304.639843280753,75.6305279269569));
#85359=CARTESIAN_POINT('Ctrl Pts',(75.2624672361846,-322.558676299804,75.6391115492116));
#85360=CARTESIAN_POINT('Ctrl Pts',(82.4798249428642,-330.212646288195,75.6771562180411));
#85361=CARTESIAN_POINT('Ctrl Pts',(98.6902707967944,-342.825622479896,75.8431732977935));
#85362=CARTESIAN_POINT('Ctrl Pts',(107.683690787476,-347.785594002476,75.9711317990764));
#85363=CARTESIAN_POINT('Ctrl Pts',(126.023069913222,-354.340138637006,76.3098567703564));
#85364=CARTESIAN_POINT('Ctrl Pts',(135.083207114917,-356.371635015224,76.501925570174));
#85365=CARTESIAN_POINT('Ctrl Pts',(148.924338523526,-357.668316903019,76.9207856483578));
#85366=CARTESIAN_POINT('Ctrl Pts',(153.579247220674,-357.810711475144,77.0819658816335));
#85367=CARTESIAN_POINT('Ctrl Pts',(160.521670574454,-357.554693148273,77.3648314770126));
#85368=CARTESIAN_POINT('Ctrl Pts',(162.82915793653,-357.391086631896,77.4659695920693));
#85369=CARTESIAN_POINT('Ctrl Pts',(167.413894984383,-356.901529412086,77.6834093931112));
#85370=CARTESIAN_POINT('Ctrl Pts',(169.690165914981,-356.571218959933,77.800168876217));
#85371=CARTESIAN_POINT('Ctrl Pts',(180.410587995582,-354.672149675074,78.3871286663314));
#85372=CARTESIAN_POINT('Ctrl Pts',(188.539471171489,-351.990508745272,78.9676971116917));
#85373=CARTESIAN_POINT('Ctrl Pts',(203.935932366808,-344.394636660447,80.2994244971851));
#85374=CARTESIAN_POINT('Ctrl Pts',(211.203510672235,-339.480369996828,81.0505889748358));
#85375=CARTESIAN_POINT('Ctrl Pts',(231.426270328895,-321.586439483533,83.4642765655722));
#85376=CARTESIAN_POINT('Ctrl Pts',(242.801650331,-305.454778835795,85.2871564557421));
#85377=CARTESIAN_POINT('Ctrl Pts',(259.787422523192,-265.857198323714,88.846412059781));
#85378=CARTESIAN_POINT('Ctrl Pts',(265.396961479631,-242.39170484102,90.582652202398));
#85379=CARTESIAN_POINT('Ctrl Pts',(269.303802179431,-189.217670775394,93.4513081720829));
#85380=CARTESIAN_POINT('Ctrl Pts',(267.601212650846,-159.509605592023,94.5836348018781));
#85381=CARTESIAN_POINT('Ctrl Pts',(260.488092878426,-122.007461671797,95.2483440922483));
#85382=CARTESIAN_POINT('Ctrl Pts',(259.365919995518,-116.723004281873,95.3235942479774));
#85383=CARTESIAN_POINT('Ctrl Pts',(256.932101050909,-106.048555274698,95.4495336771278));
#85384=CARTESIAN_POINT('Ctrl Pts',(255.614336154295,-100.659660585315,95.4992578713651));
#85385=CARTESIAN_POINT('Ctrl Pts',(251.40188561101,-84.3843231292077,95.6128833960036));
#85386=CARTESIAN_POINT('Ctrl Pts',(248.248043744655,-73.3892261805465,95.6412376442078));
#85387=CARTESIAN_POINT('Ctrl Pts',(238.097187851482,-40.3402024940961,95.6176286794984));
#85388=CARTESIAN_POINT('Ctrl Pts',(230.410833839506,-18.2225145274556,95.4569933696899));
#85389=CARTESIAN_POINT('Ctrl Pts',(201.530604066263,61.5570672312919,94.6440942086903));
#85390=CARTESIAN_POINT('Ctrl Pts',(180.38355994371,113.231534550229,93.6242109681347));
#85391=CARTESIAN_POINT('Ctrl Pts',(140.797124795906,209.938840593949,91.236348118932));
#85392=CARTESIAN_POINT('Ctrl Pts',(122.357793139117,254.971482304575,89.8683893074086));
#85393=CARTESIAN_POINT('Ctrl Pts',(90.7794276043238,345.543709944167,87.281854516083));
#85394=CARTESIAN_POINT('Ctrl Pts',(77.6398467041473,391.083508984014,86.0632256586685));
#85395=CARTESIAN_POINT('Ctrl Pts',(59.2526292615706,489.828486097094,84.2723560895427));
#85396=CARTESIAN_POINT('Ctrl Pts',(54.0050807366749,543.034307838934,83.7001064546653));
#85397=CARTESIAN_POINT('Ctrl Pts',(54.0050807343608,603.648875370191,83.7001064550861));
#85398=CARTESIAN_POINT('',(20.,-22.143643036685,76.7830741855192));
#85399=CARTESIAN_POINT('',(20.,-22.143643036685,90.7830741855191));
#85400=CARTESIAN_POINT('Origin',(20.,-22.143643036685,83.7830741855192));
#85401=CARTESIAN_POINT('',(51.7501560487334,603.648875370191,97.5173172684936));
#85402=CARTESIAN_POINT('Ctrl Pts',(20.,-22.143643036685,90.7830741855191));
#85403=CARTESIAN_POINT('Ctrl Pts',(20.0000000000198,-27.8492353264858,90.7830741857566));
#85404=CARTESIAN_POINT('Ctrl Pts',(20.016531491053,-33.4924103112104,90.7809692811259));
#85405=CARTESIAN_POINT('Ctrl Pts',(20.0854956745684,-44.652337916243,90.7729027944908));
#85406=CARTESIAN_POINT('Ctrl Pts',(20.1519455268513,-50.1688656975699,90.7669931373075));
#85407=CARTESIAN_POINT('Ctrl Pts',(20.2763301300078,-66.5284269358881,90.7436397123106));
#85408=CARTESIAN_POINT('Ctrl Pts',(20.4296113938976,-77.1799060213726,90.7200562499926));
#85409=CARTESIAN_POINT('Ctrl Pts',(21.204630097782,-108.349450811737,90.6316052988318));
#85410=CARTESIAN_POINT('Ctrl Pts',(22.10504803841,-128.083053161685,90.5490380656054));
#85411=CARTESIAN_POINT('Ctrl Pts',(26.1866133659894,-183.994412288981,90.2688168229746));
#85412=CARTESIAN_POINT('Ctrl Pts',(30.746127010843,-216.882416081384,90.0383918562974));
#85413=CARTESIAN_POINT('Ctrl Pts',(41.3926632564519,-259.039362511386,89.7639586006721));
#85414=CARTESIAN_POINT('Ctrl Pts',(45.5770679869517,-271.896024711361,89.6842863240442));
#85415=CARTESIAN_POINT('Ctrl Pts',(55.4018279120142,-295.117897261812,89.5711052176021));
#85416=CARTESIAN_POINT('Ctrl Pts',(61.0423813996187,-305.483380736572,89.537592808458));
#85417=CARTESIAN_POINT('Ctrl Pts',(73.9681096297112,-323.616276787607,89.5394453387168));
#85418=CARTESIAN_POINT('Ctrl Pts',(81.2539205629141,-331.38357033419,89.574825037295));
#85419=CARTESIAN_POINT('Ctrl Pts',(97.6502257000617,-344.201135241083,89.7372502415561));
#85420=CARTESIAN_POINT('Ctrl Pts',(106.760388060712,-349.250441287872,89.8643096573043));
#85421=CARTESIAN_POINT('Ctrl Pts',(125.319409233977,-355.926310616132,90.2023724747043));
#85422=CARTESIAN_POINT('Ctrl Pts',(134.460916219209,-357.956218127161,90.3981360471693));
#85423=CARTESIAN_POINT('Ctrl Pts',(148.381254189844,-359.260303386218,90.8193950122208));
#85424=CARTESIAN_POINT('Ctrl Pts',(153.056669136986,-359.402941416322,90.9813162075653));
#85425=CARTESIAN_POINT('Ctrl Pts',(160.021484418159,-359.146091163259,91.2650948575132));
#85426=CARTESIAN_POINT('Ctrl Pts',(162.335035463347,-358.982005239573,91.3665035078458));
#85427=CARTESIAN_POINT('Ctrl Pts',(166.929126684686,-358.491441282613,91.5843878520904));
#85428=CARTESIAN_POINT('Ctrl Pts',(169.210645617082,-358.169322998826,91.7004057485949));
#85429=CARTESIAN_POINT('Ctrl Pts',(179.919992561305,-356.169384070604,92.298422684164));
#85430=CARTESIAN_POINT('Ctrl Pts',(188.028150039962,-353.406916146197,92.886735985852));
#85431=CARTESIAN_POINT('Ctrl Pts',(203.358387400023,-345.653984304867,94.2309638137419));
#85432=CARTESIAN_POINT('Ctrl Pts',(210.580466995992,-340.663555898792,94.9868728026557));
#85433=CARTESIAN_POINT('Ctrl Pts',(230.634970522565,-322.558230840682,97.4092377737371));
#85434=CARTESIAN_POINT('Ctrl Pts',(241.855485286281,-306.310160623718,99.2301691411035));
#85435=CARTESIAN_POINT('Ctrl Pts',(258.506880498815,-266.551606234007,102.771659591371));
#85436=CARTESIAN_POINT('Ctrl Pts',(263.93861418432,-243.040695677481,104.492354248469));
#85437=CARTESIAN_POINT('Ctrl Pts',(267.516302570461,-189.829029610341,107.32426252492));
#85438=CARTESIAN_POINT('Ctrl Pts',(265.662148540819,-160.127798701236,108.435565344194));
#85439=CARTESIAN_POINT('Ctrl Pts',(258.396229893289,-122.648535323832,109.076344940978));
#85440=CARTESIAN_POINT('Ctrl Pts',(257.286143016284,-117.361163348158,109.153535727234));
#85441=CARTESIAN_POINT('Ctrl Pts',(254.851980659096,-106.685207594979,109.279492953135));
#85442=CARTESIAN_POINT('Ctrl Pts',(253.534024014268,-101.295526889627,109.329224471656));
#85443=CARTESIAN_POINT('Ctrl Pts',(249.320934663633,-85.0177209441514,109.442867244621));
#85444=CARTESIAN_POINT('Ctrl Pts',(246.16658290972,-74.0208326701545,109.471226738793));
#85445=CARTESIAN_POINT('Ctrl Pts',(236.013896109739,-40.9658464365221,109.447613584385));
#85446=CARTESIAN_POINT('Ctrl Pts',(228.325939211598,-18.8434554588877,109.28694968347));
#85447=CARTESIAN_POINT('Ctrl Pts',(199.4371324841,60.9598195272659,108.473809105488));
#85448=CARTESIAN_POINT('Ctrl Pts',(178.278774731953,112.662771270022,107.453470304555));
#85449=CARTESIAN_POINT('Ctrl Pts',(138.658245547169,209.453374230036,105.063551170246));
#85450=CARTESIAN_POINT('Ctrl Pts',(120.196014730927,254.541222475395,103.693950031325));
#85451=CARTESIAN_POINT('Ctrl Pts',(88.5733089389711,345.240633983569,101.103783619896));
#85452=CARTESIAN_POINT('Ctrl Pts',(75.4133809825114,390.851984142697,99.8832712227459));
#85453=CARTESIAN_POINT('Ctrl Pts',(57.0018485468049,489.727553050326,98.090033588344));
#85454=CARTESIAN_POINT('Ctrl Pts',(51.7501560506267,542.991128087974,97.5173172684936));
#85455=CARTESIAN_POINT('Ctrl Pts',(51.7501560487334,603.648875370191,97.5173172684936));
#85456=CARTESIAN_POINT('',(54.0050807343608,603.648875370191,83.700106455086));
#85457=CARTESIAN_POINT('Origin',(52.8776183915471,603.648875370191,90.6087118617898));
#85458=CARTESIAN_POINT('Ctrl Pts',(20.,-22.143643036685,76.7830741855192));
#85459=CARTESIAN_POINT('Ctrl Pts',(20.,-27.8457920778109,76.7830741857566));
#85460=CARTESIAN_POINT('Ctrl Pts',(20.0165214330532,-33.485592853313,76.7809705517141));
#85461=CARTESIAN_POINT('Ctrl Pts',(20.0854446608167,-44.638917128667,76.7729088380163));
#85462=CARTESIAN_POINT('Ctrl Pts',(20.1238292955523,-50.1526654673148,76.7668988331685));
#85463=CARTESIAN_POINT('Ctrl Pts',(20.4301340697073,-66.5001303791202,76.743985515181));
#85464=CARTESIAN_POINT('Ctrl Pts',(20.7188936123879,-77.141599114471,76.7227141396145));
#85465=CARTESIAN_POINT('Ctrl Pts',(21.8028495683285,-108.277666955853,76.643040982027));
#85466=CARTESIAN_POINT('Ctrl Pts',(22.8522177208893,-127.983498586547,76.568779347995));
#85467=CARTESIAN_POINT('Ctrl Pts',(27.2962882348799,-183.793342140183,76.3120470559144));
#85468=CARTESIAN_POINT('Ctrl Pts',(31.9889018993299,-216.590007789356,76.0958804243854));
#85469=CARTESIAN_POINT('Ctrl Pts',(42.752586146367,-258.54916325461,75.8385782220632));
#85470=CARTESIAN_POINT('Ctrl Pts',(46.9602598342624,-271.329384640549,75.7640306692479));
#85471=CARTESIAN_POINT('Ctrl Pts',(56.7935789905011,-294.374861216214,75.6600037328577));
#85472=CARTESIAN_POINT('Ctrl Pts',(62.4190261651095,-304.639843280753,75.6305279269569));
#85473=CARTESIAN_POINT('Ctrl Pts',(75.2624672361846,-322.558676299804,75.6391115492116));
#85474=CARTESIAN_POINT('Ctrl Pts',(82.4798249428642,-330.212646288195,75.6771562180411));
#85475=CARTESIAN_POINT('Ctrl Pts',(98.6902707967944,-342.825622479896,75.8431732977935));
#85476=CARTESIAN_POINT('Ctrl Pts',(107.683690787476,-347.785594002476,75.9711317990764));
#85477=CARTESIAN_POINT('Ctrl Pts',(126.023069913222,-354.340138637006,76.3098567703564));
#85478=CARTESIAN_POINT('Ctrl Pts',(135.083207114917,-356.371635015224,76.501925570174));
#85479=CARTESIAN_POINT('Ctrl Pts',(148.924338523526,-357.668316903019,76.9207856483578));
#85480=CARTESIAN_POINT('Ctrl Pts',(153.579247220674,-357.810711475144,77.0819658816335));
#85481=CARTESIAN_POINT('Ctrl Pts',(160.521670574454,-357.554693148273,77.3648314770126));
#85482=CARTESIAN_POINT('Ctrl Pts',(162.82915793653,-357.391086631896,77.4659695920693));
#85483=CARTESIAN_POINT('Ctrl Pts',(167.413894984383,-356.901529412086,77.6834093931112));
#85484=CARTESIAN_POINT('Ctrl Pts',(169.690165914981,-356.571218959933,77.800168876217));
#85485=CARTESIAN_POINT('Ctrl Pts',(180.410587995582,-354.672149675074,78.3871286663314));
#85486=CARTESIAN_POINT('Ctrl Pts',(188.539471171489,-351.990508745272,78.9676971116917));
#85487=CARTESIAN_POINT('Ctrl Pts',(203.935932366808,-344.394636660447,80.2994244971851));
#85488=CARTESIAN_POINT('Ctrl Pts',(211.203510672235,-339.480369996828,81.0505889748358));
#85489=CARTESIAN_POINT('Ctrl Pts',(231.426270328895,-321.586439483533,83.4642765655722));
#85490=CARTESIAN_POINT('Ctrl Pts',(242.801650331,-305.454778835795,85.2871564557421));
#85491=CARTESIAN_POINT('Ctrl Pts',(259.787422523192,-265.857198323714,88.846412059781));
#85492=CARTESIAN_POINT('Ctrl Pts',(265.396961479631,-242.39170484102,90.582652202398));
#85493=CARTESIAN_POINT('Ctrl Pts',(269.303802179431,-189.217670775394,93.4513081720829));
#85494=CARTESIAN_POINT('Ctrl Pts',(267.601212650846,-159.509605592023,94.5836348018781));
#85495=CARTESIAN_POINT('Ctrl Pts',(260.488092878426,-122.007461671797,95.2483440922483));
#85496=CARTESIAN_POINT('Ctrl Pts',(259.365919995518,-116.723004281873,95.3235942479774));
#85497=CARTESIAN_POINT('Ctrl Pts',(256.932101050909,-106.048555274698,95.4495336771278));
#85498=CARTESIAN_POINT('Ctrl Pts',(255.614336154295,-100.659660585315,95.4992578713651));
#85499=CARTESIAN_POINT('Ctrl Pts',(251.40188561101,-84.3843231292077,95.6128833960036));
#85500=CARTESIAN_POINT('Ctrl Pts',(248.248043744655,-73.3892261805465,95.6412376442078));
#85501=CARTESIAN_POINT('Ctrl Pts',(238.097187851482,-40.3402024940961,95.6176286794984));
#85502=CARTESIAN_POINT('Ctrl Pts',(230.410833839506,-18.2225145274556,95.4569933696899));
#85503=CARTESIAN_POINT('Ctrl Pts',(201.530604066263,61.5570672312919,94.6440942086903));
#85504=CARTESIAN_POINT('Ctrl Pts',(180.38355994371,113.231534550229,93.6242109681347));
#85505=CARTESIAN_POINT('Ctrl Pts',(140.797124795906,209.938840593949,91.236348118932));
#85506=CARTESIAN_POINT('Ctrl Pts',(122.357793139117,254.971482304575,89.8683893074086));
#85507=CARTESIAN_POINT('Ctrl Pts',(90.7794276043238,345.543709944167,87.281854516083));
#85508=CARTESIAN_POINT('Ctrl Pts',(77.6398467041473,391.083508984014,86.0632256586685));
#85509=CARTESIAN_POINT('Ctrl Pts',(59.2526292615706,489.828486097094,84.2723560895427));
#85510=CARTESIAN_POINT('Ctrl Pts',(54.0050807366749,543.034307838934,83.7001064546653));
#85511=CARTESIAN_POINT('Ctrl Pts',(54.0050807343608,603.648875370191,83.700106455086));
#85512=CARTESIAN_POINT('Origin',(20.,-21.143643036685,83.7830741855192));
#85513=CARTESIAN_POINT('',(20.,-21.1844254061993,74.7958939977414));
#85514=CARTESIAN_POINT('Origin',(20.,-21.1844254061993,83.7830741855192));
#85515=CARTESIAN_POINT('',(20.,-22.143643036685,75.795062050842));
#85516=CARTESIAN_POINT('Origin',(20.,-21.143643036685,75.795062050842));
#85517=CARTESIAN_POINT('Origin',(20.,-22.143643036685,83.7830741855192));
#85518=CARTESIAN_POINT('Origin',(20.,-22.143643036685,83.7830741855192));
#85519=CARTESIAN_POINT('',(20.,3.62965999324553,73.7830741855192));
#85520=CARTESIAN_POINT('Origin',(20.,3.62965999324553,83.7830741855192));
#85521=CARTESIAN_POINT('',(20.,-22.143643036685,74.8350457377612));
#85522=CARTESIAN_POINT('Origin',(20.,3.62965999324553,73.7830741855192));
#85523=CARTESIAN_POINT('Origin',(20.,-22.143643036685,83.7830741855192));
#85524=CARTESIAN_POINT('Origin',(20.,-22.143643036685,83.7830741855192));
#85525=CARTESIAN_POINT('Ctrl Pts',(20.,-22.143643036685,76.7830741855192));
#85526=CARTESIAN_POINT('Ctrl Pts',(20.,-27.8457920778109,76.7830741857566));
#85527=CARTESIAN_POINT('Ctrl Pts',(20.0165214330532,-33.485592853313,76.7809705517141));
#85528=CARTESIAN_POINT('Ctrl Pts',(20.0854446608167,-44.638917128667,76.7729088380163));
#85529=CARTESIAN_POINT('Ctrl Pts',(20.1238292955523,-50.1526654673148,76.7668988331685));
#85530=CARTESIAN_POINT('Ctrl Pts',(20.4301340697073,-66.5001303791202,76.743985515181));
#85531=CARTESIAN_POINT('Ctrl Pts',(20.7188936123879,-77.141599114471,76.7227141396145));
#85532=CARTESIAN_POINT('Ctrl Pts',(21.8028495683285,-108.277666955853,76.643040982027));
#85533=CARTESIAN_POINT('Ctrl Pts',(22.8522177208893,-127.983498586547,76.568779347995));
#85534=CARTESIAN_POINT('Ctrl Pts',(27.2962882348799,-183.793342140183,76.3120470559144));
#85535=CARTESIAN_POINT('Ctrl Pts',(31.9889018993299,-216.590007789356,76.0958804243854));
#85536=CARTESIAN_POINT('Ctrl Pts',(42.752586146367,-258.54916325461,75.8385782220632));
#85537=CARTESIAN_POINT('Ctrl Pts',(46.9602598342624,-271.329384640549,75.7640306692479));
#85538=CARTESIAN_POINT('Ctrl Pts',(56.7935789905011,-294.374861216214,75.6600037328577));
#85539=CARTESIAN_POINT('Ctrl Pts',(62.4190261651095,-304.639843280753,75.6305279269569));
#85540=CARTESIAN_POINT('Ctrl Pts',(75.2624672361846,-322.558676299804,75.6391115492116));
#85541=CARTESIAN_POINT('Ctrl Pts',(82.4798249428642,-330.212646288195,75.6771562180411));
#85542=CARTESIAN_POINT('Ctrl Pts',(98.6902707967944,-342.825622479896,75.8431732977935));
#85543=CARTESIAN_POINT('Ctrl Pts',(107.683690787476,-347.785594002476,75.9711317990764));
#85544=CARTESIAN_POINT('Ctrl Pts',(126.023069913222,-354.340138637006,76.3098567703564));
#85545=CARTESIAN_POINT('Ctrl Pts',(135.083207114917,-356.371635015224,76.501925570174));
#85546=CARTESIAN_POINT('Ctrl Pts',(148.924338523526,-357.668316903019,76.9207856483578));
#85547=CARTESIAN_POINT('Ctrl Pts',(153.579247220674,-357.810711475144,77.0819658816335));
#85548=CARTESIAN_POINT('Ctrl Pts',(160.521670574454,-357.554693148273,77.3648314770126));
#85549=CARTESIAN_POINT('Ctrl Pts',(162.82915793653,-357.391086631896,77.4659695920693));
#85550=CARTESIAN_POINT('Ctrl Pts',(167.413894984383,-356.901529412086,77.6834093931112));
#85551=CARTESIAN_POINT('Ctrl Pts',(169.690165914981,-356.571218959933,77.800168876217));
#85552=CARTESIAN_POINT('Ctrl Pts',(180.410587995582,-354.672149675074,78.3871286663314));
#85553=CARTESIAN_POINT('Ctrl Pts',(188.539471171489,-351.990508745272,78.9676971116917));
#85554=CARTESIAN_POINT('Ctrl Pts',(203.935932366808,-344.394636660447,80.2994244971851));
#85555=CARTESIAN_POINT('Ctrl Pts',(211.203510672235,-339.480369996828,81.0505889748358));
#85556=CARTESIAN_POINT('Ctrl Pts',(231.426270328895,-321.586439483533,83.4642765655722));
#85557=CARTESIAN_POINT('Ctrl Pts',(242.801650331,-305.454778835795,85.2871564557421));
#85558=CARTESIAN_POINT('Ctrl Pts',(259.787422523192,-265.857198323714,88.846412059781));
#85559=CARTESIAN_POINT('Ctrl Pts',(265.396961479631,-242.39170484102,90.582652202398));
#85560=CARTESIAN_POINT('Ctrl Pts',(269.303802179431,-189.217670775394,93.4513081720829));
#85561=CARTESIAN_POINT('Ctrl Pts',(267.601212650846,-159.509605592023,94.5836348018781));
#85562=CARTESIAN_POINT('Ctrl Pts',(260.488092878426,-122.007461671797,95.2483440922483));
#85563=CARTESIAN_POINT('Ctrl Pts',(259.365919995518,-116.723004281873,95.3235942479774));
#85564=CARTESIAN_POINT('Ctrl Pts',(256.932101050909,-106.048555274698,95.4495336771278));
#85565=CARTESIAN_POINT('Ctrl Pts',(255.614336154295,-100.659660585315,95.4992578713651));
#85566=CARTESIAN_POINT('Ctrl Pts',(251.40188561101,-84.3843231292077,95.6128833960036));
#85567=CARTESIAN_POINT('Ctrl Pts',(248.248043744655,-73.3892261805465,95.6412376442078));
#85568=CARTESIAN_POINT('Ctrl Pts',(238.097187851482,-40.3402024940961,95.6176286794984));
#85569=CARTESIAN_POINT('Ctrl Pts',(230.410833839506,-18.2225145274556,95.4569933696899));
#85570=CARTESIAN_POINT('Ctrl Pts',(201.530604066263,61.5570672312919,94.6440942086903));
#85571=CARTESIAN_POINT('Ctrl Pts',(180.38355994371,113.231534550229,93.6242109681347));
#85572=CARTESIAN_POINT('Ctrl Pts',(140.797124795906,209.938840593949,91.236348118932));
#85573=CARTESIAN_POINT('Ctrl Pts',(122.357793139117,254.971482304575,89.8683893074086));
#85574=CARTESIAN_POINT('Ctrl Pts',(90.7794276043238,345.543709944167,87.281854516083));
#85575=CARTESIAN_POINT('Ctrl Pts',(77.6398467041473,391.083508984014,86.0632256586685));
#85576=CARTESIAN_POINT('Ctrl Pts',(59.2526292615706,489.828486097094,84.2723560895427));
#85577=CARTESIAN_POINT('Ctrl Pts',(54.0050807366749,543.034307838934,83.7001064546653));
#85578=CARTESIAN_POINT('Ctrl Pts',(54.0050807343608,603.648875370191,83.7001064550861));
#85579=CARTESIAN_POINT('Ctrl Pts',(34.,-22.143643036685,76.7830741855191));
#85580=CARTESIAN_POINT('Ctrl Pts',(33.9999999999839,-27.818749567832,76.7830741857369));
#85581=CARTESIAN_POINT('Ctrl Pts',(34.0164436970964,-33.4297565255892,76.7809804490342));
#85582=CARTESIAN_POINT('Ctrl Pts',(34.0849877845006,-44.5217274543659,76.7729629323669));
#85583=CARTESIAN_POINT('Ctrl Pts',(34.1231742300284,-50.0028679006344,76.7389494577223));
#85584=CARTESIAN_POINT('Ctrl Pts',(34.4276899601393,-66.246853907463,76.8982463815691));
#85585=CARTESIAN_POINT('Ctrl Pts',(34.7126441433325,-76.8114792097519,77.0127755335157));
#85586=CARTESIAN_POINT('Ctrl Pts',(35.7801701648313,-107.689013837462,77.2436000455983));
#85587=CARTESIAN_POINT('Ctrl Pts',(36.8122807199099,-127.185635036684,77.3200887338452));
#85588=CARTESIAN_POINT('Ctrl Pts',(41.1733655791691,-182.212078558018,77.4363129347258));
#85589=CARTESIAN_POINT('Ctrl Pts',(45.7887675371877,-214.28465811726,77.3652387134946));
#85590=CARTESIAN_POINT('Ctrl Pts',(56.1071091638816,-254.559565379267,77.2809282374505));
#85591=CARTESIAN_POINT('Ctrl Pts',(60.1071507567796,-266.675138787952,77.2549720220375));
#85592=CARTESIAN_POINT('Ctrl Pts',(69.2672710615284,-288.157823623031,77.2351548953765));
#85593=CARTESIAN_POINT('Ctrl Pts',(74.4235442697514,-297.51883236657,77.241288185783));
#85594=CARTESIAN_POINT('Ctrl Pts',(85.8799878791956,-313.508885526083,77.3068472367312));
#85595=CARTESIAN_POINT('Ctrl Pts',(92.1662088124034,-320.140602612327,77.3659108227464));
#85596=CARTESIAN_POINT('Ctrl Pts',(106.074791507621,-330.965616389605,77.5558022149426));
#85597=CARTESIAN_POINT('Ctrl Pts',(113.704741593858,-335.180562056838,77.6863058336575));
#85598=CARTESIAN_POINT('Ctrl Pts',(129.547452308994,-340.84513890228,78.019344686732));
#85599=CARTESIAN_POINT('Ctrl Pts',(137.504622410254,-342.63348319117,78.1724169021146));
#85600=CARTESIAN_POINT('Ctrl Pts',(149.585403594227,-343.765248871106,78.5379883229279));
#85601=CARTESIAN_POINT('Ctrl Pts',(153.635968157751,-343.887687412075,78.6783580728553));
#85602=CARTESIAN_POINT('Ctrl Pts',(159.628436780843,-343.666700644404,78.9225120249749));
#85603=CARTESIAN_POINT('Ctrl Pts',(161.61206380368,-343.525732039158,79.0094845712665));
#85604=CARTESIAN_POINT('Ctrl Pts',(165.532545967561,-343.107103515031,79.1954129140516));
#85605=CARTESIAN_POINT('Ctrl Pts',(167.468098111069,-342.826090867219,79.3037431318874));
#85606=CARTESIAN_POINT('Ctrl Pts',(176.532101218951,-341.217569579924,79.6978427041489));
#85607=CARTESIAN_POINT('Ctrl Pts',(183.383375567806,-338.959436198211,80.1037808086076));
#85608=CARTESIAN_POINT('Ctrl Pts',(196.476071197198,-332.501375371133,81.0647133327792));
#85609=CARTESIAN_POINT('Ctrl Pts',(202.718744012329,-328.297008645753,81.6202751258499));
#85610=CARTESIAN_POINT('Ctrl Pts',(220.341909241066,-312.716811913614,83.4515942144793));
#85611=CARTESIAN_POINT('Ctrl Pts',(230.624134911047,-298.333852015906,84.8966292281925));
#85612=CARTESIAN_POINT('Ctrl Pts',(246.265932818144,-261.956042751922,87.7965104150377));
#85613=CARTESIAN_POINT('Ctrl Pts',(251.601872159868,-239.986217448384,89.2479470149237));
#85614=CARTESIAN_POINT('Ctrl Pts',(255.356970654638,-189.502920762821,91.6411093546763));
#85615=CARTESIAN_POINT('Ctrl Pts',(253.780180374585,-160.998128460726,92.5820596772374));
#85616=CARTESIAN_POINT('Ctrl Pts',(246.932276322894,-124.751374927772,93.0704364824261));
#85617=CARTESIAN_POINT('Ctrl Pts',(245.842235402124,-119.627034808441,93.1558629346225));
#85618=CARTESIAN_POINT('Ctrl Pts',(243.475097814891,-109.245042637674,93.2783520239457));
#85619=CARTESIAN_POINT('Ctrl Pts',(242.190038398626,-103.98905174219,93.3268821124474));
#85620=CARTESIAN_POINT('Ctrl Pts',(238.072169272926,-88.0791416638133,93.4379565165972));
#85621=CARTESIAN_POINT('Ctrl Pts',(234.976567368465,-77.2836801120869,93.4659513934413));
#85622=CARTESIAN_POINT('Ctrl Pts',(224.980111926361,-44.7373516402995,93.4427019766555));
#85623=CARTESIAN_POINT('Ctrl Pts',(217.369979234584,-22.8302137815567,93.2841181941716));
#85624=CARTESIAN_POINT('Ctrl Pts',(188.65251219865,56.4997474834766,92.4758003573277));
#85625=CARTESIAN_POINT('Ctrl Pts',(167.598367439946,107.953240075026,91.4612213775221));
#85626=CARTESIAN_POINT('Ctrl Pts',(128.017986339935,204.645755313006,89.0737264657378));
#85627=CARTESIAN_POINT('Ctrl Pts',(109.483389981347,249.892586601305,87.6997062527036));
#85628=CARTESIAN_POINT('Ctrl Pts',(77.5768324188997,341.406124610584,85.0862925379845));
#85629=CARTESIAN_POINT('Ctrl Pts',(64.215495896169,387.677233373842,83.8475365004758));
#85630=CARTESIAN_POINT('Ctrl Pts',(45.5165434104212,488.096320975175,82.0263070967131));
#85631=CARTESIAN_POINT('Ctrl Pts',(40.1878699233725,542.222624701163,81.4451817692483));
#85632=CARTESIAN_POINT('Ctrl Pts',(40.1878699209532,603.648875370192,81.4451817694587));
#85633=CARTESIAN_POINT('Ctrl Pts',(34.,-22.143643036685,90.7830741855191));
#85634=CARTESIAN_POINT('Ctrl Pts',(33.9999999999666,-27.822192816507,90.7830741857369));
#85635=CARTESIAN_POINT('Ctrl Pts',(34.0164537550708,-33.4365739834866,90.7809791784461));
#85636=CARTESIAN_POINT('Ctrl Pts',(34.0850387982778,-44.5351482419418,90.7729568888413));
#85637=CARTESIAN_POINT('Ctrl Pts',(34.1512904613084,-50.0190681308895,90.7390437618613));
#85638=CARTESIAN_POINT('Ctrl Pts',(34.2738860204776,-66.275150464231,90.8979005786987));
#85639=CARTESIAN_POINT('Ctrl Pts',(34.4233619248085,-76.8497861166896,91.0101176438938));
#85640=CARTESIAN_POINT('Ctrl Pts',(35.1819506943524,-107.760797693274,91.2321643624032));
#85641=CARTESIAN_POINT('Ctrl Pts',(36.0651110374872,-127.285189611952,91.3003474514556));
#85642=CARTESIAN_POINT('Ctrl Pts',(40.0636907101652,-182.413148706558,91.3930827017859));
#85643=CARTESIAN_POINT('Ctrl Pts',(44.5459926487259,-214.577066409288,91.3077501454067));
#85644=CARTESIAN_POINT('Ctrl Pts',(54.7471862739539,-255.049764636043,91.2063086160594));
#85645=CARTESIAN_POINT('Ctrl Pts',(58.7239589095343,-267.241778858765,91.1752276768338));
#85646=CARTESIAN_POINT('Ctrl Pts',(67.8755199829761,-288.900859668629,91.1462563801209));
#85647=CARTESIAN_POINT('Ctrl Pts',(73.0468995042606,-298.36236982239,91.148353067284));
#85648=CARTESIAN_POINT('Ctrl Pts',(84.5856302727223,-314.566486013887,91.2071810262364));
#85649=CARTESIAN_POINT('Ctrl Pts',(90.9403044324173,-321.311526658035,91.2635796420002));
#85650=CARTESIAN_POINT('Ctrl Pts',(105.034746410925,-332.341129151079,91.4498791587053));
#85651=CARTESIAN_POINT('Ctrl Pts',(112.781438867057,-336.645409342233,91.5794836918854));
#85652=CARTESIAN_POINT('Ctrl Pts',(128.84379162978,-342.431310881406,91.9118603910799));
#85653=CARTESIAN_POINT('Ctrl Pts',(136.882331514546,-344.218066302979,92.06862737911));
#85654=CARTESIAN_POINT('Ctrl Pts',(149.042319260545,-345.35723535437,92.4365976867908));
#85655=CARTESIAN_POINT('Ctrl Pts',(153.113390074031,-345.479917353382,92.5777083987872));
#85656=CARTESIAN_POINT('Ctrl Pts',(159.128250624564,-345.258098659325,92.8227754054756));
#85657=CARTESIAN_POINT('Ctrl Pts',(161.117941330513,-345.116650646867,92.910018487043));
#85658=CARTESIAN_POINT('Ctrl Pts',(165.047777667848,-344.697015385526,93.0963913730309));
#85659=CARTESIAN_POINT('Ctrl Pts',(166.988577813154,-344.424194906112,93.2039800042653));
#85660=CARTESIAN_POINT('Ctrl Pts',(176.041505784734,-342.714803975454,93.6091367219815));
#85661=CARTESIAN_POINT('Ctrl Pts',(182.872054436279,-340.375843599256,94.0228196827679));
#85662=CARTESIAN_POINT('Ctrl Pts',(195.898526230413,-333.760723015434,94.9962526493361));
#85663=CARTESIAN_POINT('Ctrl Pts',(202.095700336024,-329.480194547591,95.5565589536698));
#85664=CARTESIAN_POINT('Ctrl Pts',(219.550609434862,-313.688603271014,97.3965554226442));
#85665=CARTESIAN_POINT('Ctrl Pts',(229.677969866178,-299.18923380383,98.8396419135539));
#85666=CARTESIAN_POINT('Ctrl Pts',(244.985390793916,-262.650450662216,101.721757946628));
#85667=CARTESIAN_POINT('Ctrl Pts',(250.143524864557,-240.635208284846,103.157649060994));
#85668=CARTESIAN_POINT('Ctrl Pts',(253.569471045668,-190.114279597768,105.514063707513));
#85669=CARTESIAN_POINT('Ctrl Pts',(251.841116264558,-161.616321569825,106.433990219553));
#85670=CARTESIAN_POINT('Ctrl Pts',(244.840413337758,-125.392448579826,106.898437331156));
#85671=CARTESIAN_POINT('Ctrl Pts',(243.762458422889,-120.265193874764,106.985804413879));
#85672=CARTESIAN_POINT('Ctrl Pts',(241.394977423079,-109.881694957916,107.108311299953));
#85673=CARTESIAN_POINT('Ctrl Pts',(240.109726258598,-104.624918046502,107.156848712739));
#85674=CARTESIAN_POINT('Ctrl Pts',(235.991218325549,-88.712539478757,107.267940365215));
#85675=CARTESIAN_POINT('Ctrl Pts',(232.89510653369,-77.9152866016949,107.295940488026));
#85676=CARTESIAN_POINT('Ctrl Pts',(222.896820184299,-45.3629955827255,107.272686881542));
#85677=CARTESIAN_POINT('Ctrl Pts',(215.28508460652,-23.4511547129986,107.114074507951));
#85678=CARTESIAN_POINT('Ctrl Pts',(186.559040616919,55.9024997794776,106.305515254125));
#85679=CARTESIAN_POINT('Ctrl Pts',(165.493582228552,107.38447679482,105.290480713943));
#85680=CARTESIAN_POINT('Ctrl Pts',(125.879107090836,204.160288949093,102.900929517052));
#85681=CARTESIAN_POINT('Ctrl Pts',(107.321611573323,249.462326772125,101.52526697662));
#85682=CARTESIAN_POINT('Ctrl Pts',(75.3707137533804,341.103048649986,98.9082216417973));
#85683=CARTESIAN_POINT('Ctrl Pts',(61.9890301742715,387.445708532525,97.6675820645533));
#85684=CARTESIAN_POINT('Ctrl Pts',(43.265762695917,487.995387928407,95.8439845955144));
#85685=CARTESIAN_POINT('Ctrl Pts',(37.9329452373243,542.179444956935,95.2623925830766));
#85686=CARTESIAN_POINT('Ctrl Pts',(37.9329452353258,603.648875370192,95.2623925828662));
#85687=CARTESIAN_POINT('Ctrl Pts',(20.,-22.143643036685,90.7830741855191));
#85688=CARTESIAN_POINT('Ctrl Pts',(20.0000000000198,-27.8492353264858,90.7830741857566));
#85689=CARTESIAN_POINT('Ctrl Pts',(20.016531491053,-33.4924103112104,90.7809692811259));
#85690=CARTESIAN_POINT('Ctrl Pts',(20.0854956745684,-44.652337916243,90.7729027944908));
#85691=CARTESIAN_POINT('Ctrl Pts',(20.1519455268513,-50.1688656975699,90.7669931373075));
#85692=CARTESIAN_POINT('Ctrl Pts',(20.2763301300078,-66.5284269358881,90.7436397123106));
#85693=CARTESIAN_POINT('Ctrl Pts',(20.4296113938976,-77.1799060213726,90.7200562499926));
#85694=CARTESIAN_POINT('Ctrl Pts',(21.204630097782,-108.349450811737,90.6316052988318));
#85695=CARTESIAN_POINT('Ctrl Pts',(22.10504803841,-128.083053161685,90.5490380656054));
#85696=CARTESIAN_POINT('Ctrl Pts',(26.1866133659894,-183.994412288981,90.2688168229746));
#85697=CARTESIAN_POINT('Ctrl Pts',(30.746127010843,-216.882416081384,90.0383918562974));
#85698=CARTESIAN_POINT('Ctrl Pts',(41.3926632564519,-259.039362511386,89.7639586006721));
#85699=CARTESIAN_POINT('Ctrl Pts',(45.5770679869517,-271.896024711361,89.6842863240442));
#85700=CARTESIAN_POINT('Ctrl Pts',(55.4018279120142,-295.117897261812,89.5711052176021));
#85701=CARTESIAN_POINT('Ctrl Pts',(61.0423813996187,-305.483380736572,89.537592808458));
#85702=CARTESIAN_POINT('Ctrl Pts',(73.9681096297112,-323.616276787607,89.5394453387168));
#85703=CARTESIAN_POINT('Ctrl Pts',(81.2539205629141,-331.38357033419,89.574825037295));
#85704=CARTESIAN_POINT('Ctrl Pts',(97.6502257000617,-344.201135241083,89.7372502415561));
#85705=CARTESIAN_POINT('Ctrl Pts',(106.760388060712,-349.250441287872,89.8643096573043));
#85706=CARTESIAN_POINT('Ctrl Pts',(125.319409233977,-355.926310616132,90.2023724747043));
#85707=CARTESIAN_POINT('Ctrl Pts',(134.460916219209,-357.956218127161,90.3981360471693));
#85708=CARTESIAN_POINT('Ctrl Pts',(148.381254189844,-359.260303386218,90.8193950122208));
#85709=CARTESIAN_POINT('Ctrl Pts',(153.056669136986,-359.402941416322,90.9813162075653));
#85710=CARTESIAN_POINT('Ctrl Pts',(160.021484418159,-359.146091163259,91.2650948575132));
#85711=CARTESIAN_POINT('Ctrl Pts',(162.335035463347,-358.982005239573,91.3665035078458));
#85712=CARTESIAN_POINT('Ctrl Pts',(166.929126684686,-358.491441282613,91.5843878520904));
#85713=CARTESIAN_POINT('Ctrl Pts',(169.210645617082,-358.169322998826,91.7004057485949));
#85714=CARTESIAN_POINT('Ctrl Pts',(179.919992561305,-356.169384070604,92.298422684164));
#85715=CARTESIAN_POINT('Ctrl Pts',(188.028150039962,-353.406916146197,92.886735985852));
#85716=CARTESIAN_POINT('Ctrl Pts',(203.358387400023,-345.653984304867,94.2309638137419));
#85717=CARTESIAN_POINT('Ctrl Pts',(210.580466995992,-340.663555898792,94.9868728026557));
#85718=CARTESIAN_POINT('Ctrl Pts',(230.634970522565,-322.558230840682,97.4092377737371));
#85719=CARTESIAN_POINT('Ctrl Pts',(241.855485286281,-306.310160623718,99.2301691411035));
#85720=CARTESIAN_POINT('Ctrl Pts',(258.506880498815,-266.551606234007,102.771659591371));
#85721=CARTESIAN_POINT('Ctrl Pts',(263.93861418432,-243.040695677481,104.492354248469));
#85722=CARTESIAN_POINT('Ctrl Pts',(267.516302570461,-189.829029610341,107.32426252492));
#85723=CARTESIAN_POINT('Ctrl Pts',(265.662148540819,-160.127798701236,108.435565344194));
#85724=CARTESIAN_POINT('Ctrl Pts',(258.396229893289,-122.648535323832,109.076344940978));
#85725=CARTESIAN_POINT('Ctrl Pts',(257.286143016284,-117.361163348158,109.153535727234));
#85726=CARTESIAN_POINT('Ctrl Pts',(254.851980659096,-106.685207594979,109.279492953135));
#85727=CARTESIAN_POINT('Ctrl Pts',(253.534024014268,-101.295526889627,109.329224471656));
#85728=CARTESIAN_POINT('Ctrl Pts',(249.320934663633,-85.0177209441514,109.442867244621));
#85729=CARTESIAN_POINT('Ctrl Pts',(246.16658290972,-74.0208326701545,109.471226738793));
#85730=CARTESIAN_POINT('Ctrl Pts',(236.013896109739,-40.9658464365221,109.447613584385));
#85731=CARTESIAN_POINT('Ctrl Pts',(228.325939211598,-18.8434554588877,109.28694968347));
#85732=CARTESIAN_POINT('Ctrl Pts',(199.4371324841,60.9598195272659,108.473809105488));
#85733=CARTESIAN_POINT('Ctrl Pts',(178.278774731953,112.662771270022,107.453470304555));
#85734=CARTESIAN_POINT('Ctrl Pts',(138.658245547169,209.453374230036,105.063551170246));
#85735=CARTESIAN_POINT('Ctrl Pts',(120.196014730927,254.541222475395,103.693950031325));
#85736=CARTESIAN_POINT('Ctrl Pts',(88.5733089389711,345.240633983569,101.103783619896));
#85737=CARTESIAN_POINT('Ctrl Pts',(75.4133809825114,390.851984142697,99.8832712227459));
#85738=CARTESIAN_POINT('Ctrl Pts',(57.0018485468049,489.727553050326,98.090033588344));
#85739=CARTESIAN_POINT('Ctrl Pts',(51.7501560506267,542.991128087974,97.5173172684936));
#85740=CARTESIAN_POINT('Ctrl Pts',(51.7501560487334,603.648875370191,97.5173172684936));
#85741=CARTESIAN_POINT('Ctrl Pts',(6.,-22.143643036685,90.7830741855191));
#85742=CARTESIAN_POINT('Ctrl Pts',(6.00000000007298,-27.8762778364647,90.7830741857764));
#85743=CARTESIAN_POINT('Ctrl Pts',(6.01660922703522,-33.5482466389342,90.7809593838058));
#85744=CARTESIAN_POINT('Ctrl Pts',(6.08595255085911,-44.7695275905442,90.7728487001403));
#85745=CARTESIAN_POINT('Ctrl Pts',(6.15260059239406,-50.3186632642503,90.7949425127537));
#85746=CARTESIAN_POINT('Ctrl Pts',(6.27877423953789,-66.7817034075453,90.5893788459225));
#85747=CARTESIAN_POINT('Ctrl Pts',(6.43586086298679,-77.5100259260557,90.4299948560914));
#85748=CARTESIAN_POINT('Ctrl Pts',(7.22730950121153,-108.9381039302,90.0310462352604));
#85749=CARTESIAN_POINT('Ctrl Pts',(8.14498503933279,-128.880916711419,89.7977286797552));
#85750=CARTESIAN_POINT('Ctrl Pts',(12.3095360218137,-185.575675871405,89.1445509441633));
#85751=CARTESIAN_POINT('Ctrl Pts',(16.9462613729601,-219.18776575348,88.7690335671882));
#85752=CARTESIAN_POINT('Ctrl Pts',(28.0381402389499,-263.028960386728,88.3216085852849));
#85753=CARTESIAN_POINT('Ctrl Pts',(32.4301770643691,-276.550270563958,88.1933449712546));
#85754=CARTESIAN_POINT('Ctrl Pts',(42.9281358410523,-301.334934854994,87.9959540550834));
#85755=CARTESIAN_POINT('Ctrl Pts',(49.0378632949769,-312.604391650755,87.9268325496319));
#85756=CARTESIAN_POINT('Ctrl Pts',(63.3505889867002,-332.666067561327,87.8717096511972));
#85757=CARTESIAN_POINT('Ctrl Pts',(71.5675366934108,-341.455614010345,87.8860704325898));
#85758=CARTESIAN_POINT('Ctrl Pts',(90.2657049891989,-356.061141331087,88.024621324407));
#85759=CARTESIAN_POINT('Ctrl Pts',(100.739337254366,-361.85547323351,88.1491356227232));
#85760=CARTESIAN_POINT('Ctrl Pts',(121.795026838174,-369.421310350857,88.4928845583287));
#85761=CARTESIAN_POINT('Ctrl Pts',(132.039500923872,-371.694369951344,88.7276447152287));
#85762=CARTESIAN_POINT('Ctrl Pts',(147.720189119143,-373.163371418067,89.2021923376507));
#85763=CARTESIAN_POINT('Ctrl Pts',(152.999948199941,-373.325965479262,89.3849240163435));
#85764=CARTESIAN_POINT('Ctrl Pts',(160.914718211754,-373.034083667193,89.7074143095509));
#85765=CARTESIAN_POINT('Ctrl Pts',(163.552129596181,-372.84735983228,89.8229885286486));
#85766=CARTESIAN_POINT('Ctrl Pts',(168.810475701525,-372.285867179701,90.07238433115));
#85767=CARTESIAN_POINT('Ctrl Pts',(171.43271342101,-371.91445109154,90.1968314929245));
#85768=CARTESIAN_POINT('Ctrl Pts',(183.798479337875,-369.623964165754,90.9877086463466));
#85769=CARTESIAN_POINT('Ctrl Pts',(193.184245643645,-366.437988693138,91.7506522889361));
#85770=CARTESIAN_POINT('Ctrl Pts',(210.818248569633,-357.5472455943,93.4656749781478));
#85771=CARTESIAN_POINT('Ctrl Pts',(219.06523365596,-351.846917249993,94.4171866516416));
#85772=CARTESIAN_POINT('Ctrl Pts',(241.719331610269,-331.42785841035,97.42192012483));
#85773=CARTESIAN_POINT('Ctrl Pts',(254.033000706385,-313.431087443606,99.6206963686531));
#85774=CARTESIAN_POINT('Ctrl Pts',(272.028370203714,-270.452761805799,103.821561236115));
#85775=CARTESIAN_POINT('Ctrl Pts',(277.733703504083,-245.446183070117,105.827059435943));
#85776=CARTESIAN_POINT('Ctrl Pts',(281.463134095255,-189.543779622914,109.134461342326));
#85777=CARTESIAN_POINT('Ctrl Pts',(279.48318081708,-158.639275832648,110.437140468834));
#85778=CARTESIAN_POINT('Ctrl Pts',(271.952046448821,-119.904622067839,111.2542525508));
#85779=CARTESIAN_POINT('Ctrl Pts',(270.809827609678,-114.457132821552,111.321267040589));
#85780=CARTESIAN_POINT('Ctrl Pts',(268.308983895114,-103.488720232041,111.450674606317));
#85781=CARTESIAN_POINT('Ctrl Pts',(266.958321769937,-97.9661357327517,111.501600230574));
#85782=CARTESIAN_POINT('Ctrl Pts',(262.650651001717,-81.3229024095457,111.617794124028));
#85783=CARTESIAN_POINT('Ctrl Pts',(259.438059285751,-70.1263787386142,111.646512989559));
#85784=CARTESIAN_POINT('Ctrl Pts',(249.130972035179,-36.5686972903188,111.622540287227));
#85785=CARTESIAN_POINT('Ctrl Pts',(241.366793816677,-14.2357562047768,111.459824858988));
#85786=CARTESIAN_POINT('Ctrl Pts',(212.315224351282,66.0171392750542,110.64210295685));
#85787=CARTESIAN_POINT('Ctrl Pts',(191.063967235354,117.941065745225,109.616459895168));
#85788=CARTESIAN_POINT('Ctrl Pts',(151.437384003502,214.746459510979,107.22617282344));
#85789=CARTESIAN_POINT('Ctrl Pts',(133.070417888531,259.620118178664,105.86263308603));
#85790=CARTESIAN_POINT('Ctrl Pts',(101.775904124562,349.378219317153,103.299345597994));
#85791=CARTESIAN_POINT('Ctrl Pts',(88.8377317907513,394.25825975287,102.098960380939));
#85792=CARTESIAN_POINT('Ctrl Pts',(70.7379343976928,491.459718172245,100.336082581174));
#85793=CARTESIAN_POINT('Ctrl Pts',(65.5673668639291,543.802811219013,99.7722419539107));
#85794=CARTESIAN_POINT('Ctrl Pts',(65.567366862141,603.648875370191,99.772241954121));
#85795=CARTESIAN_POINT('Ctrl Pts',(6.,-22.143643036685,76.7830741855191));
#85796=CARTESIAN_POINT('Ctrl Pts',(6.00000000001608,-27.8728345877897,76.7830741857764));
#85797=CARTESIAN_POINT('Ctrl Pts',(6.01659916901003,-33.5414291810368,76.7809606543939));
#85798=CARTESIAN_POINT('Ctrl Pts',(6.08590153713278,-44.7561068029682,76.7728547436659));
#85799=CARTESIAN_POINT('Ctrl Pts',(6.12448436107623,-50.3024630339952,76.7948482086147));
#85800=CARTESIAN_POINT('Ctrl Pts',(6.43257817927521,-66.7534068507774,76.5897246487929));
#85801=CARTESIAN_POINT('Ctrl Pts',(6.72514308144325,-77.47171901919,76.4326527457133));
#85802=CARTESIAN_POINT('Ctrl Pts',(7.82552897182559,-108.866320074244,76.0424819184556));
#85803=CARTESIAN_POINT('Ctrl Pts',(8.89215472186884,-128.78136213641,75.8174699621448));
#85804=CARTESIAN_POINT('Ctrl Pts',(13.4192108905908,-185.374605722347,75.1877811771031));
#85805=CARTESIAN_POINT('Ctrl Pts',(18.189036261472,-218.895357461452,74.8265221352761));
#85806=CARTESIAN_POINT('Ctrl Pts',(29.3980631288525,-262.538761129952,74.3962282066761));
#85807=CARTESIAN_POINT('Ctrl Pts',(33.8133689117452,-275.983630493145,74.2730893164583));
#85808=CARTESIAN_POINT('Ctrl Pts',(44.3198869194738,-300.591898809396,74.0848525703389));
#85809=CARTESIAN_POINT('Ctrl Pts',(50.4145080604677,-311.760854194936,74.0197676681309));
#85810=CARTESIAN_POINT('Ctrl Pts',(64.6449465931735,-331.608467073524,73.9713758616919));
#85811=CARTESIAN_POINT('Ctrl Pts',(72.793441073325,-340.284689964064,73.9884016133359));
#85812=CARTESIAN_POINT('Ctrl Pts',(91.3057500859674,-354.685628570187,74.1305443806443));
#85813=CARTESIAN_POINT('Ctrl Pts',(101.662639981094,-360.390625948114,74.2559577644952));
#85814=CARTESIAN_POINT('Ctrl Pts',(122.498687517451,-367.835138371731,74.6003688539808));
#85815=CARTESIAN_POINT('Ctrl Pts',(132.66179181958,-370.109786839278,74.8314342382333));
#85816=CARTESIAN_POINT('Ctrl Pts',(148.263273452825,-371.571384934932,75.3035829737878));
#85817=CARTESIAN_POINT('Ctrl Pts',(153.522526283597,-371.733735538213,75.4855736904116));
#85818=CARTESIAN_POINT('Ctrl Pts',(161.414904368065,-371.442685652143,75.8071509290502));
#85819=CARTESIAN_POINT('Ctrl Pts',(164.04625206938,-371.256441224634,75.922454612872));
#85820=CARTESIAN_POINT('Ctrl Pts',(169.295244001206,-370.695955309142,76.1714058721708));
#85821=CARTESIAN_POINT('Ctrl Pts',(171.912233718893,-370.316347052647,76.2965946205466));
#85822=CARTESIAN_POINT('Ctrl Pts',(184.289074772213,-368.126729770224,77.0764146285139));
#85823=CARTESIAN_POINT('Ctrl Pts',(193.695566775172,-365.021581292332,77.8316134147758));
#85824=CARTESIAN_POINT('Ctrl Pts',(211.395793536418,-356.28789794976,79.5341356615909));
#85825=CARTESIAN_POINT('Ctrl Pts',(219.68827733214,-350.663731347904,80.4809028238217));
#85826=CARTESIAN_POINT('Ctrl Pts',(242.510631416724,-330.456067053452,83.4769589166651));
#85827=CARTESIAN_POINT('Ctrl Pts',(254.979165750953,-312.575705655683,85.6776836832917));
#85828=CARTESIAN_POINT('Ctrl Pts',(273.308912228241,-269.758353895505,89.8963137045242));
#85829=CARTESIAN_POINT('Ctrl Pts',(279.192050799395,-244.797192233655,91.9173573898723));
#85830=CARTESIAN_POINT('Ctrl Pts',(283.250633704224,-188.932420787966,95.2615069894894));
#85831=CARTESIAN_POINT('Ctrl Pts',(281.422244927106,-158.021082723321,96.5852099265189));
#85832=CARTESIAN_POINT('Ctrl Pts',(274.043909433957,-119.263548415822,97.4262517020704));
#85833=CARTESIAN_POINT('Ctrl Pts',(272.889604588913,-113.818973755306,97.4913255613324));
#85834=CARTESIAN_POINT('Ctrl Pts',(270.389104286926,-102.852067911723,97.6207153303099));
#85835=CARTESIAN_POINT('Ctrl Pts',(269.038633909964,-97.3302694284403,97.6716336302827));
#85836=CARTESIAN_POINT('Ctrl Pts',(264.731601949094,-80.689504594602,97.78781027541));
#85837=CARTESIAN_POINT('Ctrl Pts',(261.519520120845,-69.4947722490061,97.8165238949743));
#85838=CARTESIAN_POINT('Ctrl Pts',(251.214263776602,-35.9430533478927,97.7925553823412));
#85839=CARTESIAN_POINT('Ctrl Pts',(243.451688444427,-13.6148152733545,97.6298685452083));
#85840=CARTESIAN_POINT('Ctrl Pts',(214.408695933877,66.6143869791072,96.812388060053));
#85841=CARTESIAN_POINT('Ctrl Pts',(193.168752447473,118.509829025431,95.7872005587473));
#85842=CARTESIAN_POINT('Ctrl Pts',(153.576263251876,215.231925874893,93.3989697721262));
#85843=CARTESIAN_POINT('Ctrl Pts',(135.232196296888,260.050378007844,92.0370723621136));
#85844=CARTESIAN_POINT('Ctrl Pts',(103.982022789748,349.68129527775,89.4774164941815));
#85845=CARTESIAN_POINT('Ctrl Pts',(91.0641975121257,394.489784594186,88.2789148168611));
#85846=CARTESIAN_POINT('Ctrl Pts',(72.9887151127201,491.560651219013,86.5184050823723));
#85847=CARTESIAN_POINT('Ctrl Pts',(67.8222915499773,543.845990976705,85.9550311400823));
#85848=CARTESIAN_POINT('Ctrl Pts',(67.8222915477683,603.648875370191,85.9550311407135));
#85849=CARTESIAN_POINT('Ctrl Pts',(20.,-22.143643036685,76.7830741855192));
#85850=CARTESIAN_POINT('Ctrl Pts',(20.,-27.8457920778109,76.7830741857566));
#85851=CARTESIAN_POINT('Ctrl Pts',(20.0165214330532,-33.485592853313,76.7809705517141));
#85852=CARTESIAN_POINT('Ctrl Pts',(20.0854446608167,-44.638917128667,76.7729088380163));
#85853=CARTESIAN_POINT('Ctrl Pts',(20.1238292955523,-50.1526654673148,76.7668988331685));
#85854=CARTESIAN_POINT('Ctrl Pts',(20.4301340697073,-66.5001303791202,76.743985515181));
#85855=CARTESIAN_POINT('Ctrl Pts',(20.7188936123879,-77.141599114471,76.7227141396145));
#85856=CARTESIAN_POINT('Ctrl Pts',(21.8028495683285,-108.277666955853,76.643040982027));
#85857=CARTESIAN_POINT('Ctrl Pts',(22.8522177208893,-127.983498586547,76.568779347995));
#85858=CARTESIAN_POINT('Ctrl Pts',(27.2962882348799,-183.793342140183,76.3120470559144));
#85859=CARTESIAN_POINT('Ctrl Pts',(31.9889018993299,-216.590007789356,76.0958804243854));
#85860=CARTESIAN_POINT('Ctrl Pts',(42.752586146367,-258.54916325461,75.8385782220632));
#85861=CARTESIAN_POINT('Ctrl Pts',(46.9602598342624,-271.329384640549,75.7640306692479));
#85862=CARTESIAN_POINT('Ctrl Pts',(56.7935789905011,-294.374861216214,75.6600037328577));
#85863=CARTESIAN_POINT('Ctrl Pts',(62.4190261651095,-304.639843280753,75.6305279269569));
#85864=CARTESIAN_POINT('Ctrl Pts',(75.2624672361846,-322.558676299804,75.6391115492116));
#85865=CARTESIAN_POINT('Ctrl Pts',(82.4798249428642,-330.212646288195,75.6771562180411));
#85866=CARTESIAN_POINT('Ctrl Pts',(98.6902707967944,-342.825622479896,75.8431732977935));
#85867=CARTESIAN_POINT('Ctrl Pts',(107.683690787476,-347.785594002476,75.9711317990764));
#85868=CARTESIAN_POINT('Ctrl Pts',(126.023069913222,-354.340138637006,76.3098567703564));
#85869=CARTESIAN_POINT('Ctrl Pts',(135.083207114917,-356.371635015224,76.501925570174));
#85870=CARTESIAN_POINT('Ctrl Pts',(148.924338523526,-357.668316903019,76.9207856483578));
#85871=CARTESIAN_POINT('Ctrl Pts',(153.579247220674,-357.810711475144,77.0819658816335));
#85872=CARTESIAN_POINT('Ctrl Pts',(160.521670574454,-357.554693148273,77.3648314770126));
#85873=CARTESIAN_POINT('Ctrl Pts',(162.82915793653,-357.391086631896,77.4659695920693));
#85874=CARTESIAN_POINT('Ctrl Pts',(167.413894984383,-356.901529412086,77.6834093931112));
#85875=CARTESIAN_POINT('Ctrl Pts',(169.690165914981,-356.571218959933,77.800168876217));
#85876=CARTESIAN_POINT('Ctrl Pts',(180.410587995582,-354.672149675074,78.3871286663314));
#85877=CARTESIAN_POINT('Ctrl Pts',(188.539471171489,-351.990508745272,78.9676971116917));
#85878=CARTESIAN_POINT('Ctrl Pts',(203.935932366808,-344.394636660447,80.2994244971851));
#85879=CARTESIAN_POINT('Ctrl Pts',(211.203510672235,-339.480369996828,81.0505889748358));
#85880=CARTESIAN_POINT('Ctrl Pts',(231.426270328895,-321.586439483533,83.4642765655722));
#85881=CARTESIAN_POINT('Ctrl Pts',(242.801650331,-305.454778835795,85.2871564557421));
#85882=CARTESIAN_POINT('Ctrl Pts',(259.787422523192,-265.857198323714,88.846412059781));
#85883=CARTESIAN_POINT('Ctrl Pts',(265.396961479631,-242.39170484102,90.582652202398));
#85884=CARTESIAN_POINT('Ctrl Pts',(269.303802179431,-189.217670775394,93.4513081720829));
#85885=CARTESIAN_POINT('Ctrl Pts',(267.601212650846,-159.509605592023,94.5836348018781));
#85886=CARTESIAN_POINT('Ctrl Pts',(260.488092878426,-122.007461671797,95.2483440922483));
#85887=CARTESIAN_POINT('Ctrl Pts',(259.365919995518,-116.723004281873,95.3235942479774));
#85888=CARTESIAN_POINT('Ctrl Pts',(256.932101050909,-106.048555274698,95.4495336771278));
#85889=CARTESIAN_POINT('Ctrl Pts',(255.614336154295,-100.659660585315,95.4992578713651));
#85890=CARTESIAN_POINT('Ctrl Pts',(251.40188561101,-84.3843231292077,95.6128833960036));
#85891=CARTESIAN_POINT('Ctrl Pts',(248.248043744655,-73.3892261805465,95.6412376442078));
#85892=CARTESIAN_POINT('Ctrl Pts',(238.097187851482,-40.3402024940961,95.6176286794984));
#85893=CARTESIAN_POINT('Ctrl Pts',(230.410833839506,-18.2225145274556,95.4569933696899));
#85894=CARTESIAN_POINT('Ctrl Pts',(201.530604066263,61.5570672312919,94.6440942086903));
#85895=CARTESIAN_POINT('Ctrl Pts',(180.38355994371,113.231534550229,93.6242109681347));
#85896=CARTESIAN_POINT('Ctrl Pts',(140.797124795906,209.938840593949,91.236348118932));
#85897=CARTESIAN_POINT('Ctrl Pts',(122.357793139117,254.971482304575,89.8683893074086));
#85898=CARTESIAN_POINT('Ctrl Pts',(90.7794276043238,345.543709944167,87.281854516083));
#85899=CARTESIAN_POINT('Ctrl Pts',(77.6398467041473,391.083508984014,86.0632256586685));
#85900=CARTESIAN_POINT('Ctrl Pts',(59.2526292615706,489.828486097094,84.2723560895427));
#85901=CARTESIAN_POINT('Ctrl Pts',(54.0050807366749,543.034307838934,83.7001064546653));
#85902=CARTESIAN_POINT('Ctrl Pts',(54.0050807343608,603.648875370191,83.7001064550861));
#85903=CARTESIAN_POINT('Origin',(52.8776183915471,603.648875370191,90.6087118617898));
#85904=CARTESIAN_POINT('Origin',(52.8776183915471,640.125373764374,79.6087118617898));
#85905=CARTESIAN_POINT('Origin',(52.8776183915471,603.64887537019,90.6087118617898));
#130894=UNCERTAINTY_MEASURE_WITH_UNIT(LENGTH_MEASURE(0.01),#130911,
'DISTANCE_ACCURACY_VALUE',
'Maximum model space distance between geometric entities at asserted c
onnectivities');
#130900=UNCERTAINTY_MEASURE_WITH_UNIT(LENGTH_MEASURE(0.01),#130911,
'DISTANCE_ACCURACY_VALUE',
'Maximum model space distance between geometric entities at asserted c
onnectivities');
#130904=(
GEOMETRIC_REPRESENTATION_CONTEXT(3)
GLOBAL_UNCERTAINTY_ASSIGNED_CONTEXT((#130894))
GLOBAL_UNIT_ASSIGNED_CONTEXT((#130911,#130913,#130914))
REPRESENTATION_CONTEXT('','3D')
);
#130910=(
GEOMETRIC_REPRESENTATION_CONTEXT(3)
GLOBAL_UNCERTAINTY_ASSIGNED_CONTEXT((#130900))
GLOBAL_UNIT_ASSIGNED_CONTEXT((#130911,#130913,#130914))
REPRESENTATION_CONTEXT('','3D')
);
#130911=(
LENGTH_UNIT()
NAMED_UNIT(*)
SI_UNIT(.MILLI.,.METRE.)
);
#130913=(
NAMED_UNIT(*)
PLANE_ANGLE_UNIT()
SI_UNIT($,.RADIAN.)
);
#130914=(
NAMED_UNIT(*)
SI_UNIT($,.STERADIAN.)
SOLID_ANGLE_UNIT()
);
#130918=SHAPE_DEFINITION_REPRESENTATION(#130927,#130944);
#130927=PRODUCT_DEFINITION_SHAPE('',$,#130954);
#130944=SHAPE_REPRESENTATION('',(#48137),#130904);
#130950=PRODUCT_DEFINITION_CONTEXT('part definition',#130979,'design');
#130954=PRODUCT_DEFINITION('Component3','Component3',#130963,#130950);
#130963=PRODUCT_DEFINITION_FORMATION('',$,#130984);
#130979=APPLICATION_CONTEXT(
'Core Data for Automotive Mechanical Design Process');
#130980=PRODUCT_CONTEXT('part definition',#130979,'mechanical');
#130984=PRODUCT('Component3','Component3',$,(#130980));
#130991=PRESENTATION_STYLE_ASSIGNMENT((#130993));
#130993=SURFACE_STYLE_USAGE(.BOTH.,#130995);
#130995=SURFACE_SIDE_STYLE('',(#130997));
#130997=SURFACE_STYLE_FILL_AREA(#130999);
#130999=FILL_AREA_STYLE('Opaque(202,209,238)',(#131001));
#131001=FILL_AREA_STYLE_COLOUR('Opaque(202,209,238)',#131003);
#131003=COLOUR_RGB('Opaque(202,209,238)', 0.40784314, 0.44705882, 0.49803922);
ENDSEC;
END-ISO-10303-21;
